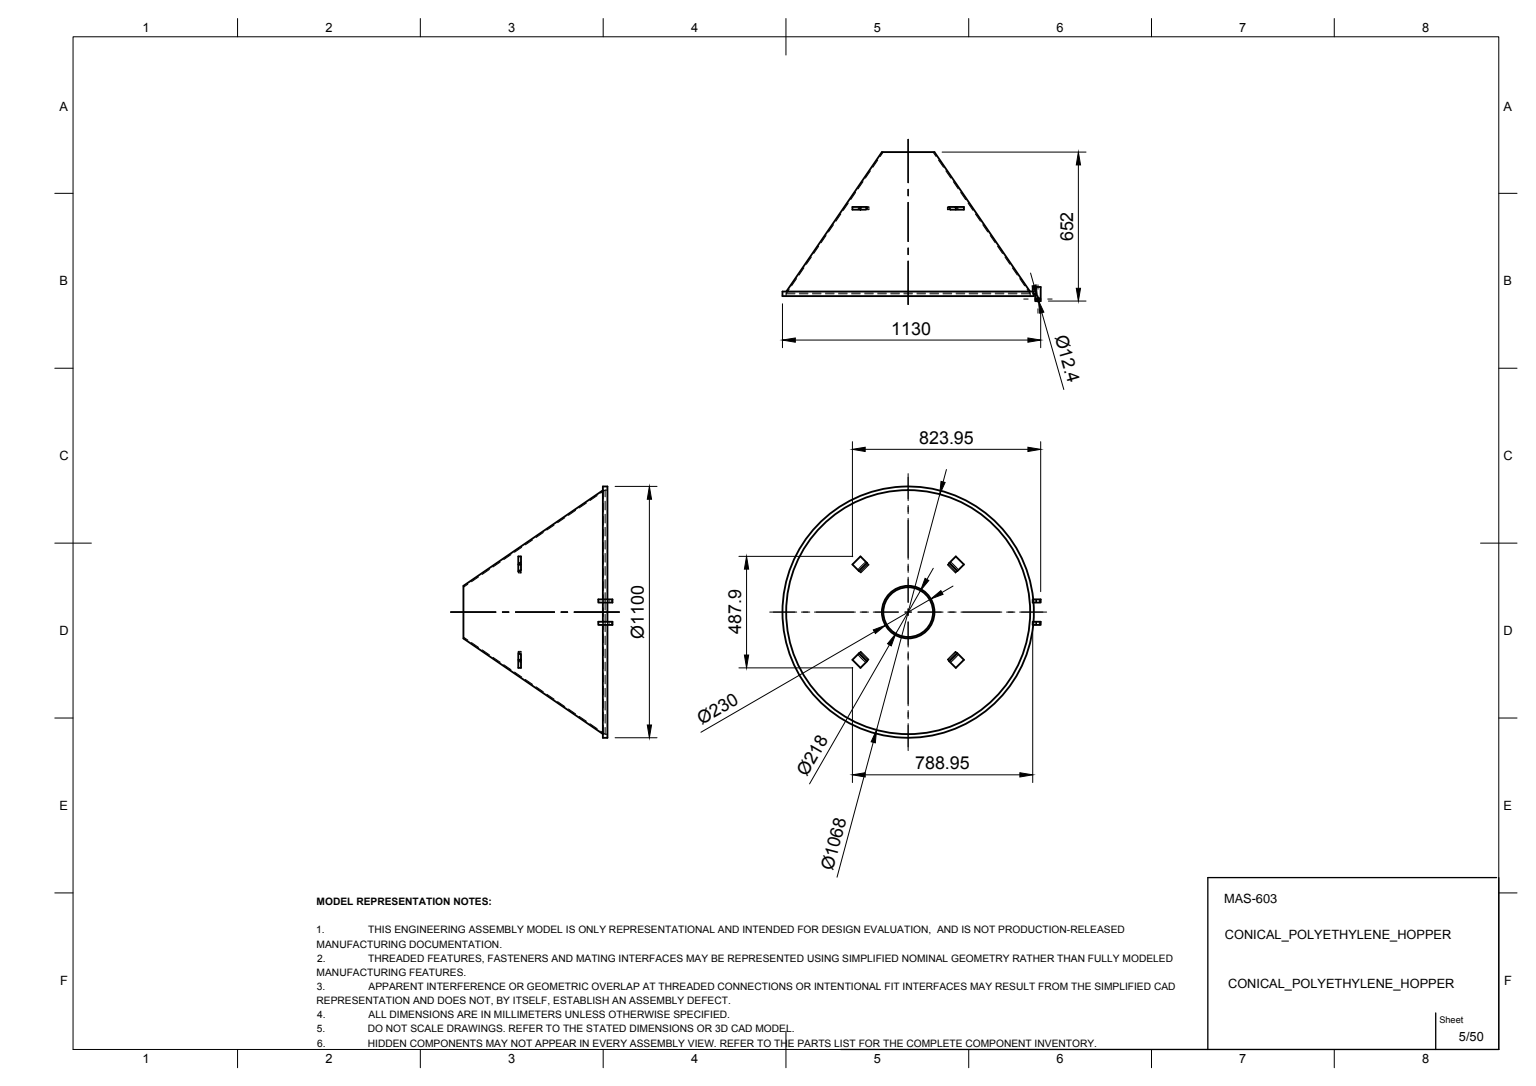
ISO-10303-21;
HEADER;
FILE_DESCRIPTION((''),'2;1');
FILE_NAME('CONICAL_POLYETHYLENE_HOPPER.step','2026-10-01T22:06:14-07:00',(''),(''),'','','');
FILE_SCHEMA (('AUTOMOTIVE_DESIGN { 1 0 10303 214 3 1 1 }'));
ENDSEC;
DATA;
#10=MECHANICAL_DESIGN_GEOMETRIC_PRESENTATION_REPRESENTATION('',(#981),#50440);
#891=SHAPE_REPRESENTATION_RELATIONSHIP('SRR','None',#50621,#936) ;
#936=ADVANCED_BREP_SHAPE_REPRESENTATION('',(#1037),#50390) ;
#981=STYLED_ITEM('',(#50884),#1037) ;
#1037=MANIFOLD_SOLID_BREP('CONICAL_POLYETHYLENE_HOPPER',#28629) ;
#1090=CONICAL_SURFACE('',#29307,32.15,0.600917014687121) ;
#1091=CONICAL_SURFACE('',#29309,32.75,0.600917014687121) ;
#1096=(
BOUNDED_CURVE()
B_SPLINE_CURVE(2,(#41351,#41352,#41353),.UNSPECIFIED.,.F.,.F.)
B_SPLINE_CURVE_WITH_KNOTS((3,3),(0.,1.45668740131038),.UNSPECIFIED.)
CURVE()
GEOMETRIC_REPRESENTATION_ITEM()
RATIONAL_B_SPLINE_CURVE((1.,1.00010597947028,1.))
REPRESENTATION_ITEM('')
) ;
#1097=(
BOUNDED_CURVE()
B_SPLINE_CURVE(2,(#41359,#41360,#41361),.UNSPECIFIED.,.F.,.F.)
B_SPLINE_CURVE_WITH_KNOTS((3,3),(0.,1.45668740131038),.UNSPECIFIED.)
CURVE()
GEOMETRIC_REPRESENTATION_ITEM()
RATIONAL_B_SPLINE_CURVE((1.,1.00010597945705,1.))
REPRESENTATION_ITEM('')
) ;
#1098=(
BOUNDED_CURVE()
B_SPLINE_CURVE(2,(#41368,#41369,#41370),.UNSPECIFIED.,.F.,.F.)
B_SPLINE_CURVE_WITH_KNOTS((3,3),(0.,1.45676753689758),.UNSPECIFIED.)
CURVE()
GEOMETRIC_REPRESENTATION_ITEM()
RATIONAL_B_SPLINE_CURVE((1.,1.00011064855622,1.))
REPRESENTATION_ITEM('')
) ;
#1099=(
BOUNDED_CURVE()
B_SPLINE_CURVE(2,(#41392,#41393,#41394),.UNSPECIFIED.,.F.,.F.)
B_SPLINE_CURVE_WITH_KNOTS((3,3),(0.,1.45676753689757),.UNSPECIFIED.)
CURVE()
GEOMETRIC_REPRESENTATION_ITEM()
RATIONAL_B_SPLINE_CURVE((1.,1.00011064897844,1.))
REPRESENTATION_ITEM('')
) ;
#1100=(
BOUNDED_CURVE()
B_SPLINE_CURVE(2,(#41409,#41410,#41411),.UNSPECIFIED.,.F.,.F.)
B_SPLINE_CURVE_WITH_KNOTS((3,3),(0.,1.45668740131038),.UNSPECIFIED.)
CURVE()
GEOMETRIC_REPRESENTATION_ITEM()
RATIONAL_B_SPLINE_CURVE((1.,1.00010597929787,1.))
REPRESENTATION_ITEM('')
) ;
#1101=(
BOUNDED_CURVE()
B_SPLINE_CURVE(2,(#41417,#41418,#41419),.UNSPECIFIED.,.F.,.F.)
B_SPLINE_CURVE_WITH_KNOTS((3,3),(0.,1.45668740131038),.UNSPECIFIED.)
CURVE()
GEOMETRIC_REPRESENTATION_ITEM()
RATIONAL_B_SPLINE_CURVE((1.,1.00010597985799,1.))
REPRESENTATION_ITEM('')
) ;
#1102=(
BOUNDED_CURVE()
B_SPLINE_CURVE(2,(#41426,#41427,#41428),.UNSPECIFIED.,.F.,.F.)
B_SPLINE_CURVE_WITH_KNOTS((3,3),(0.,1.45676753689758),.UNSPECIFIED.)
CURVE()
GEOMETRIC_REPRESENTATION_ITEM()
RATIONAL_B_SPLINE_CURVE((1.,1.00011064842347,1.))
REPRESENTATION_ITEM('')
) ;
#1103=(
BOUNDED_CURVE()
B_SPLINE_CURVE(2,(#41450,#41451,#41452),.UNSPECIFIED.,.F.,.F.)
B_SPLINE_CURVE_WITH_KNOTS((3,3),(0.,1.45676753689757),.UNSPECIFIED.)
CURVE()
GEOMETRIC_REPRESENTATION_ITEM()
RATIONAL_B_SPLINE_CURVE((1.,1.00011064825586,1.))
REPRESENTATION_ITEM('')
) ;
#1104=(
BOUNDED_CURVE()
B_SPLINE_CURVE(2,(#41467,#41468,#41469),.UNSPECIFIED.,.F.,.F.)
B_SPLINE_CURVE_WITH_KNOTS((3,3),(0.,1.45668740131038),.UNSPECIFIED.)
CURVE()
GEOMETRIC_REPRESENTATION_ITEM()
RATIONAL_B_SPLINE_CURVE((1.,1.00010597960991,1.))
REPRESENTATION_ITEM('')
) ;
#1105=(
BOUNDED_CURVE()
B_SPLINE_CURVE(2,(#41475,#41476,#41477),.UNSPECIFIED.,.F.,.F.)
B_SPLINE_CURVE_WITH_KNOTS((3,3),(0.,1.45668740131038),.UNSPECIFIED.)
CURVE()
GEOMETRIC_REPRESENTATION_ITEM()
RATIONAL_B_SPLINE_CURVE((1.,1.00010597917836,1.))
REPRESENTATION_ITEM('')
) ;
#1106=(
BOUNDED_CURVE()
B_SPLINE_CURVE(2,(#41484,#41485,#41486),.UNSPECIFIED.,.F.,.F.)
B_SPLINE_CURVE_WITH_KNOTS((3,3),(0.,1.45676753689757),.UNSPECIFIED.)
CURVE()
GEOMETRIC_REPRESENTATION_ITEM()
RATIONAL_B_SPLINE_CURVE((1.,1.00011064860079,1.))
REPRESENTATION_ITEM('')
) ;
#1107=(
BOUNDED_CURVE()
B_SPLINE_CURVE(2,(#41508,#41509,#41510),.UNSPECIFIED.,.F.,.F.)
B_SPLINE_CURVE_WITH_KNOTS((3,3),(0.,1.45676753689758),.UNSPECIFIED.)
CURVE()
GEOMETRIC_REPRESENTATION_ITEM()
RATIONAL_B_SPLINE_CURVE((1.,1.00011064816854,1.))
REPRESENTATION_ITEM('')
) ;
#1108=(
BOUNDED_CURVE()
B_SPLINE_CURVE(2,(#41525,#41526,#41527),.UNSPECIFIED.,.F.,.F.)
B_SPLINE_CURVE_WITH_KNOTS((3,3),(0.,1.45668740131038),.UNSPECIFIED.)
CURVE()
GEOMETRIC_REPRESENTATION_ITEM()
RATIONAL_B_SPLINE_CURVE((1.,1.00010597960991,1.))
REPRESENTATION_ITEM('')
) ;
#1109=(
BOUNDED_CURVE()
B_SPLINE_CURVE(2,(#41533,#41534,#41535),.UNSPECIFIED.,.F.,.F.)
B_SPLINE_CURVE_WITH_KNOTS((3,3),(0.,1.45668740131038),.UNSPECIFIED.)
CURVE()
GEOMETRIC_REPRESENTATION_ITEM()
RATIONAL_B_SPLINE_CURVE((1.,1.00010597917836,1.))
REPRESENTATION_ITEM('')
) ;
#1110=(
BOUNDED_CURVE()
B_SPLINE_CURVE(2,(#41542,#41543,#41544),.UNSPECIFIED.,.F.,.F.)
B_SPLINE_CURVE_WITH_KNOTS((3,3),(0.,1.45676753689757),.UNSPECIFIED.)
CURVE()
GEOMETRIC_REPRESENTATION_ITEM()
RATIONAL_B_SPLINE_CURVE((1.,1.00011064860079,1.))
REPRESENTATION_ITEM('')
) ;
#1111=(
BOUNDED_CURVE()
B_SPLINE_CURVE(2,(#41566,#41567,#41568),.UNSPECIFIED.,.F.,.F.)
B_SPLINE_CURVE_WITH_KNOTS((3,3),(0.,1.45676753689758),.UNSPECIFIED.)
CURVE()
GEOMETRIC_REPRESENTATION_ITEM()
RATIONAL_B_SPLINE_CURVE((1.,1.00011064816854,1.))
REPRESENTATION_ITEM('')
) ;
#1112=FACE_BOUND('',#3896,.T.) ;
#1113=FACE_BOUND('',#3903,.T.) ;
#1114=FACE_BOUND('',#3908,.T.) ;
#1115=FACE_BOUND('',#3915,.T.) ;
#1116=FACE_BOUND('',#3960,.T.) ;
#1117=FACE_BOUND('',#3962,.T.) ;
#1118=FACE_BOUND('',#3964,.T.) ;
#1119=FACE_BOUND('',#3965,.T.) ;
#1120=FACE_BOUND('',#3966,.T.) ;
#1121=FACE_BOUND('',#3967,.T.) ;
#1122=FACE_BOUND('',#3969,.T.) ;
#1123=FACE_BOUND('',#3970,.T.) ;
#1124=FACE_BOUND('',#3971,.T.) ;
#1125=FACE_BOUND('',#3972,.T.) ;
#1126=FACE_BOUND('',#3974,.T.) ;
#1408=PLANE('',#29217) ;
#1409=PLANE('',#29218) ;
#1410=PLANE('',#29219) ;
#1411=PLANE('',#29220) ;
#1412=PLANE('',#29221) ;
#1413=PLANE('',#29223) ;
#1414=PLANE('',#29224) ;
#1415=PLANE('',#29225) ;
#1416=PLANE('',#29235) ;
#1417=PLANE('',#29236) ;
#1418=PLANE('',#29237) ;
#1419=PLANE('',#29238) ;
#1420=PLANE('',#29239) ;
#1421=PLANE('',#29240) ;
#1422=PLANE('',#29241) ;
#1423=PLANE('',#29242) ;
#1424=PLANE('',#29243) ;
#1425=PLANE('',#29245) ;
#1426=PLANE('',#29246) ;
#1427=PLANE('',#29247) ;
#1428=PLANE('',#29248) ;
#1429=PLANE('',#29250) ;
#1430=PLANE('',#29252) ;
#1431=PLANE('',#29254) ;
#1432=PLANE('',#29255) ;
#1433=PLANE('',#29256) ;
#1434=PLANE('',#29257) ;
#1435=PLANE('',#29259) ;
#1436=PLANE('',#29260) ;
#1437=PLANE('',#29261) ;
#1438=PLANE('',#29262) ;
#1439=PLANE('',#29264) ;
#1440=PLANE('',#29266) ;
#1441=PLANE('',#29268) ;
#1442=PLANE('',#29269) ;
#1443=PLANE('',#29270) ;
#1444=PLANE('',#29271) ;
#1445=PLANE('',#29273) ;
#1446=PLANE('',#29274) ;
#1447=PLANE('',#29275) ;
#1448=PLANE('',#29276) ;
#1449=PLANE('',#29278) ;
#1450=PLANE('',#29280) ;
#1451=PLANE('',#29282) ;
#1452=PLANE('',#29283) ;
#1453=PLANE('',#29284) ;
#1454=PLANE('',#29285) ;
#1455=PLANE('',#29287) ;
#1456=PLANE('',#29288) ;
#1457=PLANE('',#29289) ;
#1458=PLANE('',#29290) ;
#1459=PLANE('',#29292) ;
#1460=PLANE('',#29294) ;
#1461=PLANE('',#29296) ;
#1462=PLANE('',#29297) ;
#1463=PLANE('',#29298) ;
#1464=PLANE('',#29305) ;
#1465=PLANE('',#29306) ;
#1466=PLANE('',#29311) ;
#2340=FACE_OUTER_BOUND('',#3894,.T.) ;
#2341=FACE_OUTER_BOUND('',#3895,.T.) ;
#2342=FACE_OUTER_BOUND('',#3897,.T.) ;
#2343=FACE_OUTER_BOUND('',#3898,.T.) ;
#2344=FACE_OUTER_BOUND('',#3899,.T.) ;
#2345=FACE_OUTER_BOUND('',#3900,.T.) ;
#2346=FACE_OUTER_BOUND('',#3901,.T.) ;
#2347=FACE_OUTER_BOUND('',#3902,.T.) ;
#2348=FACE_OUTER_BOUND('',#3904,.T.) ;
#2349=FACE_OUTER_BOUND('',#3905,.T.) ;
#2350=FACE_OUTER_BOUND('',#3906,.T.) ;
#2351=FACE_OUTER_BOUND('',#3907,.T.) ;
#2352=FACE_OUTER_BOUND('',#3909,.T.) ;
#2353=FACE_OUTER_BOUND('',#3910,.T.) ;
#2354=FACE_OUTER_BOUND('',#3911,.T.) ;
#2355=FACE_OUTER_BOUND('',#3912,.T.) ;
#2356=FACE_OUTER_BOUND('',#3913,.T.) ;
#2357=FACE_OUTER_BOUND('',#3914,.T.) ;
#2358=FACE_OUTER_BOUND('',#3916,.T.) ;
#2359=FACE_OUTER_BOUND('',#3917,.T.) ;
#2360=FACE_OUTER_BOUND('',#3918,.T.) ;
#2361=FACE_OUTER_BOUND('',#3919,.T.) ;
#2362=FACE_OUTER_BOUND('',#3920,.T.) ;
#2363=FACE_OUTER_BOUND('',#3921,.T.) ;
#2364=FACE_OUTER_BOUND('',#3922,.T.) ;
#2365=FACE_OUTER_BOUND('',#3923,.T.) ;
#2366=FACE_OUTER_BOUND('',#3924,.T.) ;
#2367=FACE_OUTER_BOUND('',#3925,.T.) ;
#2368=FACE_OUTER_BOUND('',#3926,.T.) ;
#2369=FACE_OUTER_BOUND('',#3927,.T.) ;
#2370=FACE_OUTER_BOUND('',#3928,.T.) ;
#2371=FACE_OUTER_BOUND('',#3929,.T.) ;
#2372=FACE_OUTER_BOUND('',#3930,.T.) ;
#2373=FACE_OUTER_BOUND('',#3931,.T.) ;
#2374=FACE_OUTER_BOUND('',#3932,.T.) ;
#2375=FACE_OUTER_BOUND('',#3933,.T.) ;
#2376=FACE_OUTER_BOUND('',#3934,.T.) ;
#2377=FACE_OUTER_BOUND('',#3935,.T.) ;
#2378=FACE_OUTER_BOUND('',#3936,.T.) ;
#2379=FACE_OUTER_BOUND('',#3937,.T.) ;
#2380=FACE_OUTER_BOUND('',#3938,.T.) ;
#2381=FACE_OUTER_BOUND('',#3939,.T.) ;
#2382=FACE_OUTER_BOUND('',#3940,.T.) ;
#2383=FACE_OUTER_BOUND('',#3941,.T.) ;
#2384=FACE_OUTER_BOUND('',#3942,.T.) ;
#2385=FACE_OUTER_BOUND('',#3943,.T.) ;
#2386=FACE_OUTER_BOUND('',#3944,.T.) ;
#2387=FACE_OUTER_BOUND('',#3945,.T.) ;
#2388=FACE_OUTER_BOUND('',#3946,.T.) ;
#2389=FACE_OUTER_BOUND('',#3947,.T.) ;
#2390=FACE_OUTER_BOUND('',#3948,.T.) ;
#2391=FACE_OUTER_BOUND('',#3949,.T.) ;
#2392=FACE_OUTER_BOUND('',#3950,.T.) ;
#2393=FACE_OUTER_BOUND('',#3951,.T.) ;
#2394=FACE_OUTER_BOUND('',#3952,.T.) ;
#2395=FACE_OUTER_BOUND('',#3953,.T.) ;
#2396=FACE_OUTER_BOUND('',#3954,.T.) ;
#2397=FACE_OUTER_BOUND('',#3955,.T.) ;
#2398=FACE_OUTER_BOUND('',#3956,.T.) ;
#2399=FACE_OUTER_BOUND('',#3957,.T.) ;
#2400=FACE_OUTER_BOUND('',#3958,.T.) ;
#2401=FACE_OUTER_BOUND('',#3959,.T.) ;
#2402=FACE_OUTER_BOUND('',#3961,.T.) ;
#2403=FACE_OUTER_BOUND('',#3963,.T.) ;
#2404=FACE_OUTER_BOUND('',#3968,.T.) ;
#2405=FACE_OUTER_BOUND('',#3973,.T.) ;
#3894=EDGE_LOOP('',(#18591,#18592,#18593,#18594)) ;
#3895=EDGE_LOOP('',(#18595,#18596,#18597,#18598,#18599,#18600,#18601,#18602)) ;
#3896=EDGE_LOOP('',(#18603)) ;
#3897=EDGE_LOOP('',(#18604,#18605,#18606,#18607)) ;
#3898=EDGE_LOOP('',(#18608,#18609,#18610,#18611)) ;
#3899=EDGE_LOOP('',(#18612,#18613,#18614,#18615)) ;
#3900=EDGE_LOOP('',(#18616,#18617,#18618,#18619)) ;
#3901=EDGE_LOOP('',(#18620,#18621,#18622,#18623)) ;
#3902=EDGE_LOOP('',(#18624,#18625,#18626,#18627,#18628,#18629,#18630,#18631)) ;
#3903=EDGE_LOOP('',(#18632)) ;
#3904=EDGE_LOOP('',(#18633,#18634,#18635,#18636)) ;
#3905=EDGE_LOOP('',(#18637,#18638,#18639,#18640,#18641,#18642,#18643,#18644,
#18645,#18646,#18647,#18648)) ;
#3906=EDGE_LOOP('',(#18649,#18650,#18651,#18652)) ;
#3907=EDGE_LOOP('',(#18653,#18654,#18655,#18656,#18657,#18658,#18659,#18660)) ;
#3908=EDGE_LOOP('',(#18661)) ;
#3909=EDGE_LOOP('',(#18662,#18663,#18664,#18665)) ;
#3910=EDGE_LOOP('',(#18666,#18667,#18668,#18669)) ;
#3911=EDGE_LOOP('',(#18670,#18671,#18672,#18673)) ;
#3912=EDGE_LOOP('',(#18674,#18675,#18676,#18677)) ;
#3913=EDGE_LOOP('',(#18678,#18679,#18680,#18681)) ;
#3914=EDGE_LOOP('',(#18682,#18683,#18684,#18685,#18686,#18687,#18688,#18689)) ;
#3915=EDGE_LOOP('',(#18690)) ;
#3916=EDGE_LOOP('',(#18691,#18692,#18693,#18694)) ;
#3917=EDGE_LOOP('',(#18695,#18696,#18697,#18698)) ;
#3918=EDGE_LOOP('',(#18699,#18700,#18701,#18702)) ;
#3919=EDGE_LOOP('',(#18703,#18704,#18705,#18706)) ;
#3920=EDGE_LOOP('',(#18707,#18708,#18709,#18710)) ;
#3921=EDGE_LOOP('',(#18711,#18712,#18713,#18714)) ;
#3922=EDGE_LOOP('',(#18715,#18716,#18717,#18718)) ;
#3923=EDGE_LOOP('',(#18719,#18720,#18721,#18722)) ;
#3924=EDGE_LOOP('',(#18723,#18724,#18725,#18726)) ;
#3925=EDGE_LOOP('',(#18727,#18728,#18729,#18730)) ;
#3926=EDGE_LOOP('',(#18731,#18732,#18733,#18734)) ;
#3927=EDGE_LOOP('',(#18735,#18736,#18737,#18738)) ;
#3928=EDGE_LOOP('',(#18739,#18740,#18741,#18742)) ;
#3929=EDGE_LOOP('',(#18743,#18744,#18745,#18746)) ;
#3930=EDGE_LOOP('',(#18747,#18748,#18749,#18750)) ;
#3931=EDGE_LOOP('',(#18751,#18752,#18753,#18754)) ;
#3932=EDGE_LOOP('',(#18755,#18756,#18757,#18758)) ;
#3933=EDGE_LOOP('',(#18759,#18760,#18761,#18762)) ;
#3934=EDGE_LOOP('',(#18763,#18764,#18765,#18766)) ;
#3935=EDGE_LOOP('',(#18767,#18768,#18769,#18770)) ;
#3936=EDGE_LOOP('',(#18771,#18772,#18773,#18774)) ;
#3937=EDGE_LOOP('',(#18775,#18776,#18777,#18778)) ;
#3938=EDGE_LOOP('',(#18779,#18780,#18781,#18782)) ;
#3939=EDGE_LOOP('',(#18783,#18784,#18785,#18786)) ;
#3940=EDGE_LOOP('',(#18787,#18788,#18789,#18790)) ;
#3941=EDGE_LOOP('',(#18791,#18792,#18793,#18794)) ;
#3942=EDGE_LOOP('',(#18795,#18796,#18797,#18798)) ;
#3943=EDGE_LOOP('',(#18799,#18800,#18801,#18802)) ;
#3944=EDGE_LOOP('',(#18803,#18804,#18805,#18806)) ;
#3945=EDGE_LOOP('',(#18807,#18808,#18809,#18810)) ;
#3946=EDGE_LOOP('',(#18811,#18812,#18813,#18814)) ;
#3947=EDGE_LOOP('',(#18815,#18816,#18817,#18818)) ;
#3948=EDGE_LOOP('',(#18819,#18820,#18821,#18822)) ;
#3949=EDGE_LOOP('',(#18823,#18824,#18825,#18826)) ;
#3950=EDGE_LOOP('',(#18827,#18828,#18829,#18830)) ;
#3951=EDGE_LOOP('',(#18831,#18832,#18833,#18834)) ;
#3952=EDGE_LOOP('',(#18835,#18836,#18837,#18838)) ;
#3953=EDGE_LOOP('',(#18839,#18840,#18841,#18842)) ;
#3954=EDGE_LOOP('',(#18843,#18844,#18845,#18846)) ;
#3955=EDGE_LOOP('',(#18847,#18848,#18849,#18850)) ;
#3956=EDGE_LOOP('',(#18851,#18852,#18853,#18854)) ;
#3957=EDGE_LOOP('',(#18855,#18856,#18857,#18858)) ;
#3958=EDGE_LOOP('',(#18859,#18860,#18861,#18862)) ;
#3959=EDGE_LOOP('',(#18863,#18864,#18865,#18866,#18867,#18868,#18869,#18870,
#18871)) ;
#3960=EDGE_LOOP('',(#18872)) ;
#3961=EDGE_LOOP('',(#18873)) ;
#3962=EDGE_LOOP('',(#18874)) ;
#3963=EDGE_LOOP('',(#18875,#18876,#18877,#18878)) ;
#3964=EDGE_LOOP('',(#18879,#18880,#18881,#18882)) ;
#3965=EDGE_LOOP('',(#18883,#18884,#18885,#18886)) ;
#3966=EDGE_LOOP('',(#18887,#18888,#18889,#18890)) ;
#3967=EDGE_LOOP('',(#18891,#18892,#18893,#18894)) ;
#3968=EDGE_LOOP('',(#18895,#18896,#18897,#18898)) ;
#3969=EDGE_LOOP('',(#18899,#18900,#18901,#18902)) ;
#3970=EDGE_LOOP('',(#18903,#18904,#18905,#18906)) ;
#3971=EDGE_LOOP('',(#18907,#18908,#18909,#18910)) ;
#3972=EDGE_LOOP('',(#18911,#18912,#18913,#18914)) ;
#3973=EDGE_LOOP('',(#18915)) ;
#3974=EDGE_LOOP('',(#18916)) ;
#5744=LINE('',#41230,#8216) ;
#5745=LINE('',#41235,#8217) ;
#5746=LINE('',#41237,#8218) ;
#5747=LINE('',#41239,#8219) ;
#5748=LINE('',#41241,#8220) ;
#5749=LINE('',#41243,#8221) ;
#5750=LINE('',#41245,#8222) ;
#5751=LINE('',#41247,#8223) ;
#5752=LINE('',#41248,#8224) ;
#5753=LINE('',#41251,#8225) ;
#5754=LINE('',#41253,#8226) ;
#5755=LINE('',#41254,#8227) ;
#5756=LINE('',#41257,#8228) ;
#5757=LINE('',#41259,#8229) ;
#5758=LINE('',#41260,#8230) ;
#5759=LINE('',#41263,#8231) ;
#5760=LINE('',#41264,#8232) ;
#5761=LINE('',#41268,#8233) ;
#5762=LINE('',#41271,#8234) ;
#5763=LINE('',#41272,#8235) ;
#5764=LINE('',#41275,#8236) ;
#5765=LINE('',#41276,#8237) ;
#5766=LINE('',#41277,#8238) ;
#5767=LINE('',#41283,#8239) ;
#5768=LINE('',#41287,#8240) ;
#5769=LINE('',#41291,#8241) ;
#5770=LINE('',#41298,#8242) ;
#5771=LINE('',#41302,#8243) ;
#5772=LINE('',#41304,#8244) ;
#5773=LINE('',#41306,#8245) ;
#5774=LINE('',#41308,#8246) ;
#5775=LINE('',#41310,#8247) ;
#5776=LINE('',#41312,#8248) ;
#5777=LINE('',#41313,#8249) ;
#5778=LINE('',#41316,#8250) ;
#5779=LINE('',#41318,#8251) ;
#5780=LINE('',#41319,#8252) ;
#5781=LINE('',#41322,#8253) ;
#5782=LINE('',#41324,#8254) ;
#5783=LINE('',#41325,#8255) ;
#5784=LINE('',#41328,#8256) ;
#5785=LINE('',#41329,#8257) ;
#5786=LINE('',#41331,#8258) ;
#5787=LINE('',#41334,#8259) ;
#5788=LINE('',#41335,#8260) ;
#5789=LINE('',#41337,#8261) ;
#5790=LINE('',#41338,#8262) ;
#5791=LINE('',#41345,#8263) ;
#5792=LINE('',#41347,#8264) ;
#5793=LINE('',#41348,#8265) ;
#5794=LINE('',#41355,#8266) ;
#5795=LINE('',#41356,#8267) ;
#5796=LINE('',#41363,#8268) ;
#5797=LINE('',#41364,#8269) ;
#5798=LINE('',#41372,#8270) ;
#5799=LINE('',#41374,#8271) ;
#5800=LINE('',#41375,#8272) ;
#5801=LINE('',#41378,#8273) ;
#5802=LINE('',#41383,#8274) ;
#5803=LINE('',#41384,#8275) ;
#5804=LINE('',#41389,#8276) ;
#5805=LINE('',#41390,#8277) ;
#5806=LINE('',#41395,#8278) ;
#5807=LINE('',#41403,#8279) ;
#5808=LINE('',#41405,#8280) ;
#5809=LINE('',#41406,#8281) ;
#5810=LINE('',#41413,#8282) ;
#5811=LINE('',#41414,#8283) ;
#5812=LINE('',#41421,#8284) ;
#5813=LINE('',#41422,#8285) ;
#5814=LINE('',#41430,#8286) ;
#5815=LINE('',#41432,#8287) ;
#5816=LINE('',#41433,#8288) ;
#5817=LINE('',#41436,#8289) ;
#5818=LINE('',#41441,#8290) ;
#5819=LINE('',#41442,#8291) ;
#5820=LINE('',#41447,#8292) ;
#5821=LINE('',#41448,#8293) ;
#5822=LINE('',#41453,#8294) ;
#5823=LINE('',#41461,#8295) ;
#5824=LINE('',#41463,#8296) ;
#5825=LINE('',#41464,#8297) ;
#5826=LINE('',#41471,#8298) ;
#5827=LINE('',#41472,#8299) ;
#5828=LINE('',#41479,#8300) ;
#5829=LINE('',#41480,#8301) ;
#5830=LINE('',#41488,#8302) ;
#5831=LINE('',#41490,#8303) ;
#5832=LINE('',#41491,#8304) ;
#5833=LINE('',#41494,#8305) ;
#5834=LINE('',#41499,#8306) ;
#5835=LINE('',#41500,#8307) ;
#5836=LINE('',#41505,#8308) ;
#5837=LINE('',#41506,#8309) ;
#5838=LINE('',#41511,#8310) ;
#5839=LINE('',#41519,#8311) ;
#5840=LINE('',#41521,#8312) ;
#5841=LINE('',#41522,#8313) ;
#5842=LINE('',#41529,#8314) ;
#5843=LINE('',#41530,#8315) ;
#5844=LINE('',#41537,#8316) ;
#5845=LINE('',#41538,#8317) ;
#5846=LINE('',#41546,#8318) ;
#5847=LINE('',#41548,#8319) ;
#5848=LINE('',#41549,#8320) ;
#5849=LINE('',#41552,#8321) ;
#5850=LINE('',#41557,#8322) ;
#5851=LINE('',#41558,#8323) ;
#5852=LINE('',#41563,#8324) ;
#5853=LINE('',#41564,#8325) ;
#5854=LINE('',#41569,#8326) ;
#5855=LINE('',#41576,#8327) ;
#5856=LINE('',#41582,#8328) ;
#5857=LINE('',#41589,#8329) ;
#5858=LINE('',#41592,#8330) ;
#8216=VECTOR('',#32401,0.62) ;
#8217=VECTOR('',#32406,1.) ;
#8218=VECTOR('',#32407,1.) ;
#8219=VECTOR('',#32408,1.) ;
#8220=VECTOR('',#32409,1.) ;
#8221=VECTOR('',#32410,1.) ;
#8222=VECTOR('',#32411,1.) ;
#8223=VECTOR('',#32412,1.) ;
#8224=VECTOR('',#32413,1.) ;
#8225=VECTOR('',#32416,1.) ;
#8226=VECTOR('',#32417,1.) ;
#8227=VECTOR('',#32418,1.) ;
#8228=VECTOR('',#32421,1.) ;
#8229=VECTOR('',#32422,1.) ;
#8230=VECTOR('',#32423,1.) ;
#8231=VECTOR('',#32426,1.) ;
#8232=VECTOR('',#32427,1.) ;
#8233=VECTOR('',#32432,1.) ;
#8234=VECTOR('',#32435,1.) ;
#8235=VECTOR('',#32436,1.) ;
#8236=VECTOR('',#32439,1.) ;
#8237=VECTOR('',#32440,1.) ;
#8238=VECTOR('',#32441,1.) ;
#8239=VECTOR('',#32448,55.) ;
#8240=VECTOR('',#32451,1.) ;
#8241=VECTOR('',#32454,1.) ;
#8242=VECTOR('',#32463,0.62) ;
#8243=VECTOR('',#32468,1.) ;
#8244=VECTOR('',#32469,1.) ;
#8245=VECTOR('',#32470,1.) ;
#8246=VECTOR('',#32471,1.) ;
#8247=VECTOR('',#32472,1.) ;
#8248=VECTOR('',#32473,1.) ;
#8249=VECTOR('',#32474,1.) ;
#8250=VECTOR('',#32477,1.) ;
#8251=VECTOR('',#32478,1.) ;
#8252=VECTOR('',#32479,1.) ;
#8253=VECTOR('',#32482,1.) ;
#8254=VECTOR('',#32483,1.) ;
#8255=VECTOR('',#32484,1.) ;
#8256=VECTOR('',#32487,1.) ;
#8257=VECTOR('',#32488,1.) ;
#8258=VECTOR('',#32491,1.) ;
#8259=VECTOR('',#32494,1.) ;
#8260=VECTOR('',#32495,1.) ;
#8261=VECTOR('',#32498,1.) ;
#8262=VECTOR('',#32499,1.) ;
#8263=VECTOR('',#32506,1.) ;
#8264=VECTOR('',#32507,1.) ;
#8265=VECTOR('',#32508,1.) ;
#8266=VECTOR('',#32511,1.) ;
#8267=VECTOR('',#32512,1.) ;
#8268=VECTOR('',#32515,1.) ;
#8269=VECTOR('',#32516,1.) ;
#8270=VECTOR('',#32519,1.) ;
#8271=VECTOR('',#32520,1.) ;
#8272=VECTOR('',#32521,1.) ;
#8273=VECTOR('',#32526,1.) ;
#8274=VECTOR('',#32531,1.) ;
#8275=VECTOR('',#32532,1.) ;
#8276=VECTOR('',#32537,1.) ;
#8277=VECTOR('',#32538,1.) ;
#8278=VECTOR('',#32541,1.) ;
#8279=VECTOR('',#32550,1.) ;
#8280=VECTOR('',#32551,1.) ;
#8281=VECTOR('',#32552,1.) ;
#8282=VECTOR('',#32555,1.) ;
#8283=VECTOR('',#32556,1.) ;
#8284=VECTOR('',#32559,1.) ;
#8285=VECTOR('',#32560,1.) ;
#8286=VECTOR('',#32563,1.) ;
#8287=VECTOR('',#32564,1.) ;
#8288=VECTOR('',#32565,1.) ;
#8289=VECTOR('',#32570,1.) ;
#8290=VECTOR('',#32575,1.) ;
#8291=VECTOR('',#32576,1.) ;
#8292=VECTOR('',#32581,1.) ;
#8293=VECTOR('',#32582,1.) ;
#8294=VECTOR('',#32585,1.) ;
#8295=VECTOR('',#32594,1.) ;
#8296=VECTOR('',#32595,1.) ;
#8297=VECTOR('',#32596,1.) ;
#8298=VECTOR('',#32599,1.) ;
#8299=VECTOR('',#32600,1.) ;
#8300=VECTOR('',#32603,1.) ;
#8301=VECTOR('',#32604,1.) ;
#8302=VECTOR('',#32607,1.) ;
#8303=VECTOR('',#32608,1.) ;
#8304=VECTOR('',#32609,1.) ;
#8305=VECTOR('',#32614,1.) ;
#8306=VECTOR('',#32619,1.) ;
#8307=VECTOR('',#32620,1.) ;
#8308=VECTOR('',#32625,1.) ;
#8309=VECTOR('',#32626,1.) ;
#8310=VECTOR('',#32629,1.) ;
#8311=VECTOR('',#32638,1.) ;
#8312=VECTOR('',#32639,1.) ;
#8313=VECTOR('',#32640,1.) ;
#8314=VECTOR('',#32643,1.) ;
#8315=VECTOR('',#32644,1.) ;
#8316=VECTOR('',#32647,1.) ;
#8317=VECTOR('',#32648,1.) ;
#8318=VECTOR('',#32651,1.) ;
#8319=VECTOR('',#32652,1.) ;
#8320=VECTOR('',#32653,1.) ;
#8321=VECTOR('',#32658,1.) ;
#8322=VECTOR('',#32663,1.) ;
#8323=VECTOR('',#32664,1.) ;
#8324=VECTOR('',#32669,1.) ;
#8325=VECTOR('',#32670,1.) ;
#8326=VECTOR('',#32673,1.) ;
#8327=VECTOR('',#32682,53.4) ;
#8328=VECTOR('',#32689,53.4) ;
#8329=VECTOR('',#32700,32.15) ;
#8330=VECTOR('',#32703,32.75) ;
#10688=CIRCLE('',#29215,0.62) ;
#10689=CIRCLE('',#29216,0.62) ;
#10690=CIRCLE('',#29222,55.) ;
#10691=CIRCLE('',#29227,55.) ;
#10692=CIRCLE('',#29228,55.) ;
#10693=CIRCLE('',#29229,55.) ;
#10694=CIRCLE('',#29230,55.) ;
#10695=CIRCLE('',#29231,55.) ;
#10696=CIRCLE('',#29233,0.62) ;
#10697=CIRCLE('',#29234,0.62) ;
#10698=CIRCLE('',#29244,28.7741935483871) ;
#10699=CIRCLE('',#29249,27.9516129032258) ;
#10700=CIRCLE('',#29251,27.3516129032258) ;
#10701=CIRCLE('',#29253,28.1741935483871) ;
#10702=CIRCLE('',#29258,28.7741935483871) ;
#10703=CIRCLE('',#29263,27.9516129032258) ;
#10704=CIRCLE('',#29265,27.3516129032258) ;
#10705=CIRCLE('',#29267,28.1741935483871) ;
#10706=CIRCLE('',#29272,28.7741935483871) ;
#10707=CIRCLE('',#29277,27.9516129032258) ;
#10708=CIRCLE('',#29279,27.3516129032258) ;
#10709=CIRCLE('',#29281,28.1741935483871) ;
#10710=CIRCLE('',#29286,28.7741935483871) ;
#10711=CIRCLE('',#29291,27.9516129032258) ;
#10712=CIRCLE('',#29293,27.3516129032258) ;
#10713=CIRCLE('',#29295,28.1741935483871) ;
#10714=CIRCLE('',#29300,53.4) ;
#10715=CIRCLE('',#29301,53.4) ;
#10716=CIRCLE('',#29303,53.4) ;
#10717=CIRCLE('',#29304,53.4) ;
#10718=CIRCLE('',#29308,10.9) ;
#10719=CIRCLE('',#29310,11.5) ;
#11855=VERTEX_POINT('',#41227) ;
#11856=VERTEX_POINT('',#41229) ;
#11857=VERTEX_POINT('',#41233) ;
#11858=VERTEX_POINT('',#41234) ;
#11859=VERTEX_POINT('',#41236) ;
#11860=VERTEX_POINT('',#41238) ;
#11861=VERTEX_POINT('',#41240) ;
#11862=VERTEX_POINT('',#41242) ;
#11863=VERTEX_POINT('',#41244) ;
#11864=VERTEX_POINT('',#41246) ;
#11865=VERTEX_POINT('',#41250) ;
#11866=VERTEX_POINT('',#41252) ;
#11867=VERTEX_POINT('',#41256) ;
#11868=VERTEX_POINT('',#41258) ;
#11869=VERTEX_POINT('',#41262) ;
#11870=VERTEX_POINT('',#41266) ;
#11871=VERTEX_POINT('',#41270) ;
#11872=VERTEX_POINT('',#41274) ;
#11873=VERTEX_POINT('',#41280) ;
#11874=VERTEX_POINT('',#41282) ;
#11875=VERTEX_POINT('',#41284) ;
#11876=VERTEX_POINT('',#41286) ;
#11877=VERTEX_POINT('',#41288) ;
#11878=VERTEX_POINT('',#41290) ;
#11879=VERTEX_POINT('',#41295) ;
#11880=VERTEX_POINT('',#41297) ;
#11881=VERTEX_POINT('',#41301) ;
#11882=VERTEX_POINT('',#41303) ;
#11883=VERTEX_POINT('',#41305) ;
#11884=VERTEX_POINT('',#41307) ;
#11885=VERTEX_POINT('',#41309) ;
#11886=VERTEX_POINT('',#41311) ;
#11887=VERTEX_POINT('',#41315) ;
#11888=VERTEX_POINT('',#41317) ;
#11889=VERTEX_POINT('',#41321) ;
#11890=VERTEX_POINT('',#41323) ;
#11891=VERTEX_POINT('',#41327) ;
#11892=VERTEX_POINT('',#41333) ;
#11893=VERTEX_POINT('',#41341) ;
#11894=VERTEX_POINT('',#41342) ;
#11895=VERTEX_POINT('',#41344) ;
#11896=VERTEX_POINT('',#41346) ;
#11897=VERTEX_POINT('',#41350) ;
#11898=VERTEX_POINT('',#41354) ;
#11899=VERTEX_POINT('',#41358) ;
#11900=VERTEX_POINT('',#41362) ;
#11901=VERTEX_POINT('',#41366) ;
#11902=VERTEX_POINT('',#41367) ;
#11903=VERTEX_POINT('',#41371) ;
#11904=VERTEX_POINT('',#41373) ;
#11905=VERTEX_POINT('',#41380) ;
#11906=VERTEX_POINT('',#41382) ;
#11907=VERTEX_POINT('',#41386) ;
#11908=VERTEX_POINT('',#41388) ;
#11909=VERTEX_POINT('',#41399) ;
#11910=VERTEX_POINT('',#41400) ;
#11911=VERTEX_POINT('',#41402) ;
#11912=VERTEX_POINT('',#41404) ;
#11913=VERTEX_POINT('',#41408) ;
#11914=VERTEX_POINT('',#41412) ;
#11915=VERTEX_POINT('',#41416) ;
#11916=VERTEX_POINT('',#41420) ;
#11917=VERTEX_POINT('',#41424) ;
#11918=VERTEX_POINT('',#41425) ;
#11919=VERTEX_POINT('',#41429) ;
#11920=VERTEX_POINT('',#41431) ;
#11921=VERTEX_POINT('',#41438) ;
#11922=VERTEX_POINT('',#41440) ;
#11923=VERTEX_POINT('',#41444) ;
#11924=VERTEX_POINT('',#41446) ;
#11925=VERTEX_POINT('',#41457) ;
#11926=VERTEX_POINT('',#41458) ;
#11927=VERTEX_POINT('',#41460) ;
#11928=VERTEX_POINT('',#41462) ;
#11929=VERTEX_POINT('',#41466) ;
#11930=VERTEX_POINT('',#41470) ;
#11931=VERTEX_POINT('',#41474) ;
#11932=VERTEX_POINT('',#41478) ;
#11933=VERTEX_POINT('',#41482) ;
#11934=VERTEX_POINT('',#41483) ;
#11935=VERTEX_POINT('',#41487) ;
#11936=VERTEX_POINT('',#41489) ;
#11937=VERTEX_POINT('',#41496) ;
#11938=VERTEX_POINT('',#41498) ;
#11939=VERTEX_POINT('',#41502) ;
#11940=VERTEX_POINT('',#41504) ;
#11941=VERTEX_POINT('',#41515) ;
#11942=VERTEX_POINT('',#41516) ;
#11943=VERTEX_POINT('',#41518) ;
#11944=VERTEX_POINT('',#41520) ;
#11945=VERTEX_POINT('',#41524) ;
#11946=VERTEX_POINT('',#41528) ;
#11947=VERTEX_POINT('',#41532) ;
#11948=VERTEX_POINT('',#41536) ;
#11949=VERTEX_POINT('',#41540) ;
#11950=VERTEX_POINT('',#41541) ;
#11951=VERTEX_POINT('',#41545) ;
#11952=VERTEX_POINT('',#41547) ;
#11953=VERTEX_POINT('',#41554) ;
#11954=VERTEX_POINT('',#41556) ;
#11955=VERTEX_POINT('',#41560) ;
#11956=VERTEX_POINT('',#41562) ;
#11957=VERTEX_POINT('',#41573) ;
#11958=VERTEX_POINT('',#41575) ;
#11959=VERTEX_POINT('',#41579) ;
#11960=VERTEX_POINT('',#41581) ;
#11961=VERTEX_POINT('',#41587) ;
#11962=VERTEX_POINT('',#41591) ;
#14561=EDGE_CURVE('',#11855,#11855,#10688,.T.) ;
#14562=EDGE_CURVE('',#11855,#11856,#5744,.T.) ;
#14563=EDGE_CURVE('',#11856,#11856,#10689,.T.) ;
#14564=EDGE_CURVE('',#11857,#11858,#5745,.T.) ;
#14565=EDGE_CURVE('',#11859,#11857,#5746,.T.) ;
#14566=EDGE_CURVE('',#11859,#11860,#5747,.T.) ;
#14567=EDGE_CURVE('',#11861,#11860,#5748,.T.) ;
#14568=EDGE_CURVE('',#11862,#11861,#5749,.T.) ;
#14569=EDGE_CURVE('',#11863,#11862,#5750,.T.) ;
#14570=EDGE_CURVE('',#11863,#11864,#5751,.T.) ;
#14571=EDGE_CURVE('',#11858,#11864,#5752,.T.) ;
#14572=EDGE_CURVE('',#11865,#11859,#5753,.T.) ;
#14573=EDGE_CURVE('',#11865,#11866,#5754,.T.) ;
#14574=EDGE_CURVE('',#11860,#11866,#5755,.T.) ;
#14575=EDGE_CURVE('',#11862,#11867,#5756,.T.) ;
#14576=EDGE_CURVE('',#11867,#11868,#5757,.T.) ;
#14577=EDGE_CURVE('',#11868,#11863,#5758,.T.) ;
#14578=EDGE_CURVE('',#11868,#11869,#5759,.T.) ;
#14579=EDGE_CURVE('',#11864,#11869,#5760,.T.) ;
#14580=EDGE_CURVE('',#11858,#11870,#10690,.T.) ;
#14581=EDGE_CURVE('',#11869,#11870,#5761,.T.) ;
#14582=EDGE_CURVE('',#11866,#11871,#5762,.T.) ;
#14583=EDGE_CURVE('',#11871,#11861,#5763,.T.) ;
#14584=EDGE_CURVE('',#11870,#11872,#5764,.T.) ;
#14585=EDGE_CURVE('',#11867,#11871,#5765,.T.) ;
#14586=EDGE_CURVE('',#11872,#11865,#5766,.T.) ;
#14587=EDGE_CURVE('',#11873,#11873,#10691,.T.) ;
#14588=EDGE_CURVE('',#11873,#11874,#5767,.T.) ;
#14589=EDGE_CURVE('',#11875,#11874,#10692,.T.) ;
#14590=EDGE_CURVE('',#11875,#11876,#5768,.T.) ;
#14591=EDGE_CURVE('',#11876,#11877,#10693,.T.) ;
#14592=EDGE_CURVE('',#11877,#11878,#5769,.T.) ;
#14593=EDGE_CURVE('',#11857,#11878,#10694,.T.) ;
#14594=EDGE_CURVE('',#11874,#11872,#10695,.T.) ;
#14595=EDGE_CURVE('',#11879,#11879,#10696,.T.) ;
#14596=EDGE_CURVE('',#11879,#11880,#5770,.T.) ;
#14597=EDGE_CURVE('',#11880,#11880,#10697,.T.) ;
#14598=EDGE_CURVE('',#11881,#11875,#5771,.T.) ;
#14599=EDGE_CURVE('',#11881,#11882,#5772,.T.) ;
#14600=EDGE_CURVE('',#11883,#11882,#5773,.T.) ;
#14601=EDGE_CURVE('',#11884,#11883,#5774,.T.) ;
#14602=EDGE_CURVE('',#11885,#11884,#5775,.T.) ;
#14603=EDGE_CURVE('',#11885,#11886,#5776,.T.) ;
#14604=EDGE_CURVE('',#11876,#11886,#5777,.T.) ;
#14605=EDGE_CURVE('',#11887,#11881,#5778,.T.) ;
#14606=EDGE_CURVE('',#11887,#11888,#5779,.T.) ;
#14607=EDGE_CURVE('',#11882,#11888,#5780,.T.) ;
#14608=EDGE_CURVE('',#11884,#11889,#5781,.T.) ;
#14609=EDGE_CURVE('',#11889,#11890,#5782,.T.) ;
#14610=EDGE_CURVE('',#11890,#11885,#5783,.T.) ;
#14611=EDGE_CURVE('',#11890,#11891,#5784,.T.) ;
#14612=EDGE_CURVE('',#11886,#11891,#5785,.T.) ;
#14613=EDGE_CURVE('',#11891,#11877,#5786,.T.) ;
#14614=EDGE_CURVE('',#11888,#11892,#5787,.T.) ;
#14615=EDGE_CURVE('',#11892,#11883,#5788,.T.) ;
#14616=EDGE_CURVE('',#11889,#11892,#5789,.T.) ;
#14617=EDGE_CURVE('',#11878,#11887,#5790,.T.) ;
#14618=EDGE_CURVE('',#11893,#11894,#10698,.T.) ;
#14619=EDGE_CURVE('',#11893,#11895,#5791,.T.) ;
#14620=EDGE_CURVE('',#11895,#11896,#5792,.T.) ;
#14621=EDGE_CURVE('',#11896,#11894,#5793,.T.) ;
#14622=EDGE_CURVE('',#11897,#11893,#1096,.T.) ;
#14623=EDGE_CURVE('',#11898,#11897,#5794,.T.) ;
#14624=EDGE_CURVE('',#11895,#11898,#5795,.T.) ;
#14625=EDGE_CURVE('',#11894,#11899,#1097,.T.) ;
#14626=EDGE_CURVE('',#11896,#11900,#5796,.T.) ;
#14627=EDGE_CURVE('',#11899,#11900,#5797,.T.) ;
#14628=EDGE_CURVE('',#11901,#11902,#1098,.T.) ;
#14629=EDGE_CURVE('',#11903,#11901,#5798,.T.) ;
#14630=EDGE_CURVE('',#11904,#11903,#5799,.T.) ;
#14631=EDGE_CURVE('',#11902,#11904,#5800,.T.) ;
#14632=EDGE_CURVE('',#11899,#11897,#10699,.T.) ;
#14633=EDGE_CURVE('',#11900,#11898,#5801,.T.) ;
#14634=EDGE_CURVE('',#11905,#11901,#10700,.T.) ;
#14635=EDGE_CURVE('',#11905,#11906,#5802,.T.) ;
#14636=EDGE_CURVE('',#11906,#11903,#5803,.T.) ;
#14637=EDGE_CURVE('',#11902,#11907,#10701,.T.) ;
#14638=EDGE_CURVE('',#11904,#11908,#5804,.T.) ;
#14639=EDGE_CURVE('',#11908,#11907,#5805,.T.) ;
#14640=EDGE_CURVE('',#11907,#11905,#1099,.T.) ;
#14641=EDGE_CURVE('',#11908,#11906,#5806,.T.) ;
#14642=EDGE_CURVE('',#11909,#11910,#10702,.T.) ;
#14643=EDGE_CURVE('',#11909,#11911,#5807,.T.) ;
#14644=EDGE_CURVE('',#11911,#11912,#5808,.T.) ;
#14645=EDGE_CURVE('',#11912,#11910,#5809,.T.) ;
#14646=EDGE_CURVE('',#11913,#11909,#1100,.T.) ;
#14647=EDGE_CURVE('',#11914,#11913,#5810,.T.) ;
#14648=EDGE_CURVE('',#11911,#11914,#5811,.T.) ;
#14649=EDGE_CURVE('',#11910,#11915,#1101,.T.) ;
#14650=EDGE_CURVE('',#11912,#11916,#5812,.T.) ;
#14651=EDGE_CURVE('',#11915,#11916,#5813,.T.) ;
#14652=EDGE_CURVE('',#11917,#11918,#1102,.T.) ;
#14653=EDGE_CURVE('',#11919,#11917,#5814,.T.) ;
#14654=EDGE_CURVE('',#11920,#11919,#5815,.T.) ;
#14655=EDGE_CURVE('',#11918,#11920,#5816,.T.) ;
#14656=EDGE_CURVE('',#11915,#11913,#10703,.T.) ;
#14657=EDGE_CURVE('',#11916,#11914,#5817,.T.) ;
#14658=EDGE_CURVE('',#11921,#11917,#10704,.T.) ;
#14659=EDGE_CURVE('',#11921,#11922,#5818,.T.) ;
#14660=EDGE_CURVE('',#11922,#11919,#5819,.T.) ;
#14661=EDGE_CURVE('',#11918,#11923,#10705,.T.) ;
#14662=EDGE_CURVE('',#11920,#11924,#5820,.T.) ;
#14663=EDGE_CURVE('',#11924,#11923,#5821,.T.) ;
#14664=EDGE_CURVE('',#11923,#11921,#1103,.T.) ;
#14665=EDGE_CURVE('',#11924,#11922,#5822,.T.) ;
#14666=EDGE_CURVE('',#11925,#11926,#10706,.T.) ;
#14667=EDGE_CURVE('',#11925,#11927,#5823,.T.) ;
#14668=EDGE_CURVE('',#11927,#11928,#5824,.T.) ;
#14669=EDGE_CURVE('',#11928,#11926,#5825,.T.) ;
#14670=EDGE_CURVE('',#11929,#11925,#1104,.T.) ;
#14671=EDGE_CURVE('',#11930,#11929,#5826,.T.) ;
#14672=EDGE_CURVE('',#11927,#11930,#5827,.T.) ;
#14673=EDGE_CURVE('',#11926,#11931,#1105,.T.) ;
#14674=EDGE_CURVE('',#11928,#11932,#5828,.T.) ;
#14675=EDGE_CURVE('',#11931,#11932,#5829,.T.) ;
#14676=EDGE_CURVE('',#11933,#11934,#1106,.T.) ;
#14677=EDGE_CURVE('',#11935,#11933,#5830,.T.) ;
#14678=EDGE_CURVE('',#11936,#11935,#5831,.T.) ;
#14679=EDGE_CURVE('',#11934,#11936,#5832,.T.) ;
#14680=EDGE_CURVE('',#11931,#11929,#10707,.T.) ;
#14681=EDGE_CURVE('',#11932,#11930,#5833,.T.) ;
#14682=EDGE_CURVE('',#11937,#11933,#10708,.T.) ;
#14683=EDGE_CURVE('',#11937,#11938,#5834,.T.) ;
#14684=EDGE_CURVE('',#11938,#11935,#5835,.T.) ;
#14685=EDGE_CURVE('',#11934,#11939,#10709,.T.) ;
#14686=EDGE_CURVE('',#11936,#11940,#5836,.T.) ;
#14687=EDGE_CURVE('',#11940,#11939,#5837,.T.) ;
#14688=EDGE_CURVE('',#11939,#11937,#1107,.T.) ;
#14689=EDGE_CURVE('',#11940,#11938,#5838,.T.) ;
#14690=EDGE_CURVE('',#11941,#11942,#10710,.T.) ;
#14691=EDGE_CURVE('',#11941,#11943,#5839,.T.) ;
#14692=EDGE_CURVE('',#11943,#11944,#5840,.T.) ;
#14693=EDGE_CURVE('',#11944,#11942,#5841,.T.) ;
#14694=EDGE_CURVE('',#11945,#11941,#1108,.T.) ;
#14695=EDGE_CURVE('',#11946,#11945,#5842,.T.) ;
#14696=EDGE_CURVE('',#11943,#11946,#5843,.T.) ;
#14697=EDGE_CURVE('',#11942,#11947,#1109,.T.) ;
#14698=EDGE_CURVE('',#11944,#11948,#5844,.T.) ;
#14699=EDGE_CURVE('',#11947,#11948,#5845,.T.) ;
#14700=EDGE_CURVE('',#11949,#11950,#1110,.T.) ;
#14701=EDGE_CURVE('',#11951,#11949,#5846,.T.) ;
#14702=EDGE_CURVE('',#11952,#11951,#5847,.T.) ;
#14703=EDGE_CURVE('',#11950,#11952,#5848,.T.) ;
#14704=EDGE_CURVE('',#11947,#11945,#10711,.T.) ;
#14705=EDGE_CURVE('',#11948,#11946,#5849,.T.) ;
#14706=EDGE_CURVE('',#11953,#11949,#10712,.T.) ;
#14707=EDGE_CURVE('',#11953,#11954,#5850,.T.) ;
#14708=EDGE_CURVE('',#11954,#11951,#5851,.T.) ;
#14709=EDGE_CURVE('',#11950,#11955,#10713,.T.) ;
#14710=EDGE_CURVE('',#11952,#11956,#5852,.T.) ;
#14711=EDGE_CURVE('',#11956,#11955,#5853,.T.) ;
#14712=EDGE_CURVE('',#11955,#11953,#1111,.T.) ;
#14713=EDGE_CURVE('',#11956,#11954,#5854,.T.) ;
#14714=EDGE_CURVE('',#11957,#11957,#10714,.T.) ;
#14715=EDGE_CURVE('',#11957,#11958,#5855,.T.) ;
#14716=EDGE_CURVE('',#11958,#11958,#10715,.T.) ;
#14717=EDGE_CURVE('',#11959,#11959,#10716,.T.) ;
#14718=EDGE_CURVE('',#11959,#11960,#5856,.T.) ;
#14719=EDGE_CURVE('',#11960,#11960,#10717,.T.) ;
#14720=EDGE_CURVE('',#11961,#11961,#10718,.T.) ;
#14721=EDGE_CURVE('',#11961,#11959,#5857,.T.) ;
#14722=EDGE_CURVE('',#11958,#11962,#5858,.T.) ;
#14723=EDGE_CURVE('',#11962,#11962,#10719,.T.) ;
#18591=ORIENTED_EDGE('',*,*,#14561,.F.) ;
#18592=ORIENTED_EDGE('',*,*,#14562,.T.) ;
#18593=ORIENTED_EDGE('',*,*,#14563,.F.) ;
#18594=ORIENTED_EDGE('',*,*,#14562,.F.) ;
#18595=ORIENTED_EDGE('',*,*,#14564,.F.) ;
#18596=ORIENTED_EDGE('',*,*,#14565,.F.) ;
#18597=ORIENTED_EDGE('',*,*,#14566,.T.) ;
#18598=ORIENTED_EDGE('',*,*,#14567,.F.) ;
#18599=ORIENTED_EDGE('',*,*,#14568,.F.) ;
#18600=ORIENTED_EDGE('',*,*,#14569,.F.) ;
#18601=ORIENTED_EDGE('',*,*,#14570,.T.) ;
#18602=ORIENTED_EDGE('',*,*,#14571,.F.) ;
#18603=ORIENTED_EDGE('',*,*,#14561,.T.) ;
#18604=ORIENTED_EDGE('',*,*,#14572,.F.) ;
#18605=ORIENTED_EDGE('',*,*,#14573,.T.) ;
#18606=ORIENTED_EDGE('',*,*,#14574,.F.) ;
#18607=ORIENTED_EDGE('',*,*,#14566,.F.) ;
#18608=ORIENTED_EDGE('',*,*,#14569,.T.) ;
#18609=ORIENTED_EDGE('',*,*,#14575,.T.) ;
#18610=ORIENTED_EDGE('',*,*,#14576,.T.) ;
#18611=ORIENTED_EDGE('',*,*,#14577,.T.) ;
#18612=ORIENTED_EDGE('',*,*,#14578,.T.) ;
#18613=ORIENTED_EDGE('',*,*,#14579,.F.) ;
#18614=ORIENTED_EDGE('',*,*,#14570,.F.) ;
#18615=ORIENTED_EDGE('',*,*,#14577,.F.) ;
#18616=ORIENTED_EDGE('',*,*,#14580,.F.) ;
#18617=ORIENTED_EDGE('',*,*,#14571,.T.) ;
#18618=ORIENTED_EDGE('',*,*,#14579,.T.) ;
#18619=ORIENTED_EDGE('',*,*,#14581,.T.) ;
#18620=ORIENTED_EDGE('',*,*,#14567,.T.) ;
#18621=ORIENTED_EDGE('',*,*,#14574,.T.) ;
#18622=ORIENTED_EDGE('',*,*,#14582,.T.) ;
#18623=ORIENTED_EDGE('',*,*,#14583,.T.) ;
#18624=ORIENTED_EDGE('',*,*,#14584,.F.) ;
#18625=ORIENTED_EDGE('',*,*,#14581,.F.) ;
#18626=ORIENTED_EDGE('',*,*,#14578,.F.) ;
#18627=ORIENTED_EDGE('',*,*,#14576,.F.) ;
#18628=ORIENTED_EDGE('',*,*,#14585,.T.) ;
#18629=ORIENTED_EDGE('',*,*,#14582,.F.) ;
#18630=ORIENTED_EDGE('',*,*,#14573,.F.) ;
#18631=ORIENTED_EDGE('',*,*,#14586,.F.) ;
#18632=ORIENTED_EDGE('',*,*,#14563,.T.) ;
#18633=ORIENTED_EDGE('',*,*,#14568,.T.) ;
#18634=ORIENTED_EDGE('',*,*,#14583,.F.) ;
#18635=ORIENTED_EDGE('',*,*,#14585,.F.) ;
#18636=ORIENTED_EDGE('',*,*,#14575,.F.) ;
#18637=ORIENTED_EDGE('',*,*,#14587,.F.) ;
#18638=ORIENTED_EDGE('',*,*,#14588,.T.) ;
#18639=ORIENTED_EDGE('',*,*,#14589,.F.) ;
#18640=ORIENTED_EDGE('',*,*,#14590,.T.) ;
#18641=ORIENTED_EDGE('',*,*,#14591,.T.) ;
#18642=ORIENTED_EDGE('',*,*,#14592,.T.) ;
#18643=ORIENTED_EDGE('',*,*,#14593,.F.) ;
#18644=ORIENTED_EDGE('',*,*,#14564,.T.) ;
#18645=ORIENTED_EDGE('',*,*,#14580,.T.) ;
#18646=ORIENTED_EDGE('',*,*,#14584,.T.) ;
#18647=ORIENTED_EDGE('',*,*,#14594,.F.) ;
#18648=ORIENTED_EDGE('',*,*,#14588,.F.) ;
#18649=ORIENTED_EDGE('',*,*,#14595,.F.) ;
#18650=ORIENTED_EDGE('',*,*,#14596,.T.) ;
#18651=ORIENTED_EDGE('',*,*,#14597,.F.) ;
#18652=ORIENTED_EDGE('',*,*,#14596,.F.) ;
#18653=ORIENTED_EDGE('',*,*,#14590,.F.) ;
#18654=ORIENTED_EDGE('',*,*,#14598,.F.) ;
#18655=ORIENTED_EDGE('',*,*,#14599,.T.) ;
#18656=ORIENTED_EDGE('',*,*,#14600,.F.) ;
#18657=ORIENTED_EDGE('',*,*,#14601,.F.) ;
#18658=ORIENTED_EDGE('',*,*,#14602,.F.) ;
#18659=ORIENTED_EDGE('',*,*,#14603,.T.) ;
#18660=ORIENTED_EDGE('',*,*,#14604,.F.) ;
#18661=ORIENTED_EDGE('',*,*,#14597,.T.) ;
#18662=ORIENTED_EDGE('',*,*,#14605,.F.) ;
#18663=ORIENTED_EDGE('',*,*,#14606,.T.) ;
#18664=ORIENTED_EDGE('',*,*,#14607,.F.) ;
#18665=ORIENTED_EDGE('',*,*,#14599,.F.) ;
#18666=ORIENTED_EDGE('',*,*,#14602,.T.) ;
#18667=ORIENTED_EDGE('',*,*,#14608,.T.) ;
#18668=ORIENTED_EDGE('',*,*,#14609,.T.) ;
#18669=ORIENTED_EDGE('',*,*,#14610,.T.) ;
#18670=ORIENTED_EDGE('',*,*,#14611,.T.) ;
#18671=ORIENTED_EDGE('',*,*,#14612,.F.) ;
#18672=ORIENTED_EDGE('',*,*,#14603,.F.) ;
#18673=ORIENTED_EDGE('',*,*,#14610,.F.) ;
#18674=ORIENTED_EDGE('',*,*,#14591,.F.) ;
#18675=ORIENTED_EDGE('',*,*,#14604,.T.) ;
#18676=ORIENTED_EDGE('',*,*,#14612,.T.) ;
#18677=ORIENTED_EDGE('',*,*,#14613,.T.) ;
#18678=ORIENTED_EDGE('',*,*,#14600,.T.) ;
#18679=ORIENTED_EDGE('',*,*,#14607,.T.) ;
#18680=ORIENTED_EDGE('',*,*,#14614,.T.) ;
#18681=ORIENTED_EDGE('',*,*,#14615,.T.) ;
#18682=ORIENTED_EDGE('',*,*,#14592,.F.) ;
#18683=ORIENTED_EDGE('',*,*,#14613,.F.) ;
#18684=ORIENTED_EDGE('',*,*,#14611,.F.) ;
#18685=ORIENTED_EDGE('',*,*,#14609,.F.) ;
#18686=ORIENTED_EDGE('',*,*,#14616,.T.) ;
#18687=ORIENTED_EDGE('',*,*,#14614,.F.) ;
#18688=ORIENTED_EDGE('',*,*,#14606,.F.) ;
#18689=ORIENTED_EDGE('',*,*,#14617,.F.) ;
#18690=ORIENTED_EDGE('',*,*,#14595,.T.) ;
#18691=ORIENTED_EDGE('',*,*,#14601,.T.) ;
#18692=ORIENTED_EDGE('',*,*,#14615,.F.) ;
#18693=ORIENTED_EDGE('',*,*,#14616,.F.) ;
#18694=ORIENTED_EDGE('',*,*,#14608,.F.) ;
#18695=ORIENTED_EDGE('',*,*,#14618,.F.) ;
#18696=ORIENTED_EDGE('',*,*,#14619,.T.) ;
#18697=ORIENTED_EDGE('',*,*,#14620,.T.) ;
#18698=ORIENTED_EDGE('',*,*,#14621,.T.) ;
#18699=ORIENTED_EDGE('',*,*,#14622,.F.) ;
#18700=ORIENTED_EDGE('',*,*,#14623,.F.) ;
#18701=ORIENTED_EDGE('',*,*,#14624,.F.) ;
#18702=ORIENTED_EDGE('',*,*,#14619,.F.) ;
#18703=ORIENTED_EDGE('',*,*,#14625,.F.) ;
#18704=ORIENTED_EDGE('',*,*,#14621,.F.) ;
#18705=ORIENTED_EDGE('',*,*,#14626,.T.) ;
#18706=ORIENTED_EDGE('',*,*,#14627,.F.) ;
#18707=ORIENTED_EDGE('',*,*,#14628,.F.) ;
#18708=ORIENTED_EDGE('',*,*,#14629,.F.) ;
#18709=ORIENTED_EDGE('',*,*,#14630,.F.) ;
#18710=ORIENTED_EDGE('',*,*,#14631,.F.) ;
#18711=ORIENTED_EDGE('',*,*,#14632,.F.) ;
#18712=ORIENTED_EDGE('',*,*,#14627,.T.) ;
#18713=ORIENTED_EDGE('',*,*,#14633,.T.) ;
#18714=ORIENTED_EDGE('',*,*,#14623,.T.) ;
#18715=ORIENTED_EDGE('',*,*,#14634,.F.) ;
#18716=ORIENTED_EDGE('',*,*,#14635,.T.) ;
#18717=ORIENTED_EDGE('',*,*,#14636,.T.) ;
#18718=ORIENTED_EDGE('',*,*,#14629,.T.) ;
#18719=ORIENTED_EDGE('',*,*,#14637,.F.) ;
#18720=ORIENTED_EDGE('',*,*,#14631,.T.) ;
#18721=ORIENTED_EDGE('',*,*,#14638,.T.) ;
#18722=ORIENTED_EDGE('',*,*,#14639,.T.) ;
#18723=ORIENTED_EDGE('',*,*,#14640,.F.) ;
#18724=ORIENTED_EDGE('',*,*,#14639,.F.) ;
#18725=ORIENTED_EDGE('',*,*,#14641,.T.) ;
#18726=ORIENTED_EDGE('',*,*,#14635,.F.) ;
#18727=ORIENTED_EDGE('',*,*,#14630,.T.) ;
#18728=ORIENTED_EDGE('',*,*,#14636,.F.) ;
#18729=ORIENTED_EDGE('',*,*,#14641,.F.) ;
#18730=ORIENTED_EDGE('',*,*,#14638,.F.) ;
#18731=ORIENTED_EDGE('',*,*,#14624,.T.) ;
#18732=ORIENTED_EDGE('',*,*,#14633,.F.) ;
#18733=ORIENTED_EDGE('',*,*,#14626,.F.) ;
#18734=ORIENTED_EDGE('',*,*,#14620,.F.) ;
#18735=ORIENTED_EDGE('',*,*,#14642,.F.) ;
#18736=ORIENTED_EDGE('',*,*,#14643,.T.) ;
#18737=ORIENTED_EDGE('',*,*,#14644,.T.) ;
#18738=ORIENTED_EDGE('',*,*,#14645,.T.) ;
#18739=ORIENTED_EDGE('',*,*,#14646,.F.) ;
#18740=ORIENTED_EDGE('',*,*,#14647,.F.) ;
#18741=ORIENTED_EDGE('',*,*,#14648,.F.) ;
#18742=ORIENTED_EDGE('',*,*,#14643,.F.) ;
#18743=ORIENTED_EDGE('',*,*,#14649,.F.) ;
#18744=ORIENTED_EDGE('',*,*,#14645,.F.) ;
#18745=ORIENTED_EDGE('',*,*,#14650,.T.) ;
#18746=ORIENTED_EDGE('',*,*,#14651,.F.) ;
#18747=ORIENTED_EDGE('',*,*,#14652,.F.) ;
#18748=ORIENTED_EDGE('',*,*,#14653,.F.) ;
#18749=ORIENTED_EDGE('',*,*,#14654,.F.) ;
#18750=ORIENTED_EDGE('',*,*,#14655,.F.) ;
#18751=ORIENTED_EDGE('',*,*,#14656,.F.) ;
#18752=ORIENTED_EDGE('',*,*,#14651,.T.) ;
#18753=ORIENTED_EDGE('',*,*,#14657,.T.) ;
#18754=ORIENTED_EDGE('',*,*,#14647,.T.) ;
#18755=ORIENTED_EDGE('',*,*,#14658,.F.) ;
#18756=ORIENTED_EDGE('',*,*,#14659,.T.) ;
#18757=ORIENTED_EDGE('',*,*,#14660,.T.) ;
#18758=ORIENTED_EDGE('',*,*,#14653,.T.) ;
#18759=ORIENTED_EDGE('',*,*,#14661,.F.) ;
#18760=ORIENTED_EDGE('',*,*,#14655,.T.) ;
#18761=ORIENTED_EDGE('',*,*,#14662,.T.) ;
#18762=ORIENTED_EDGE('',*,*,#14663,.T.) ;
#18763=ORIENTED_EDGE('',*,*,#14664,.F.) ;
#18764=ORIENTED_EDGE('',*,*,#14663,.F.) ;
#18765=ORIENTED_EDGE('',*,*,#14665,.T.) ;
#18766=ORIENTED_EDGE('',*,*,#14659,.F.) ;
#18767=ORIENTED_EDGE('',*,*,#14654,.T.) ;
#18768=ORIENTED_EDGE('',*,*,#14660,.F.) ;
#18769=ORIENTED_EDGE('',*,*,#14665,.F.) ;
#18770=ORIENTED_EDGE('',*,*,#14662,.F.) ;
#18771=ORIENTED_EDGE('',*,*,#14648,.T.) ;
#18772=ORIENTED_EDGE('',*,*,#14657,.F.) ;
#18773=ORIENTED_EDGE('',*,*,#14650,.F.) ;
#18774=ORIENTED_EDGE('',*,*,#14644,.F.) ;
#18775=ORIENTED_EDGE('',*,*,#14666,.F.) ;
#18776=ORIENTED_EDGE('',*,*,#14667,.T.) ;
#18777=ORIENTED_EDGE('',*,*,#14668,.T.) ;
#18778=ORIENTED_EDGE('',*,*,#14669,.T.) ;
#18779=ORIENTED_EDGE('',*,*,#14670,.F.) ;
#18780=ORIENTED_EDGE('',*,*,#14671,.F.) ;
#18781=ORIENTED_EDGE('',*,*,#14672,.F.) ;
#18782=ORIENTED_EDGE('',*,*,#14667,.F.) ;
#18783=ORIENTED_EDGE('',*,*,#14673,.F.) ;
#18784=ORIENTED_EDGE('',*,*,#14669,.F.) ;
#18785=ORIENTED_EDGE('',*,*,#14674,.T.) ;
#18786=ORIENTED_EDGE('',*,*,#14675,.F.) ;
#18787=ORIENTED_EDGE('',*,*,#14676,.F.) ;
#18788=ORIENTED_EDGE('',*,*,#14677,.F.) ;
#18789=ORIENTED_EDGE('',*,*,#14678,.F.) ;
#18790=ORIENTED_EDGE('',*,*,#14679,.F.) ;
#18791=ORIENTED_EDGE('',*,*,#14680,.F.) ;
#18792=ORIENTED_EDGE('',*,*,#14675,.T.) ;
#18793=ORIENTED_EDGE('',*,*,#14681,.T.) ;
#18794=ORIENTED_EDGE('',*,*,#14671,.T.) ;
#18795=ORIENTED_EDGE('',*,*,#14682,.F.) ;
#18796=ORIENTED_EDGE('',*,*,#14683,.T.) ;
#18797=ORIENTED_EDGE('',*,*,#14684,.T.) ;
#18798=ORIENTED_EDGE('',*,*,#14677,.T.) ;
#18799=ORIENTED_EDGE('',*,*,#14685,.F.) ;
#18800=ORIENTED_EDGE('',*,*,#14679,.T.) ;
#18801=ORIENTED_EDGE('',*,*,#14686,.T.) ;
#18802=ORIENTED_EDGE('',*,*,#14687,.T.) ;
#18803=ORIENTED_EDGE('',*,*,#14688,.F.) ;
#18804=ORIENTED_EDGE('',*,*,#14687,.F.) ;
#18805=ORIENTED_EDGE('',*,*,#14689,.T.) ;
#18806=ORIENTED_EDGE('',*,*,#14683,.F.) ;
#18807=ORIENTED_EDGE('',*,*,#14678,.T.) ;
#18808=ORIENTED_EDGE('',*,*,#14684,.F.) ;
#18809=ORIENTED_EDGE('',*,*,#14689,.F.) ;
#18810=ORIENTED_EDGE('',*,*,#14686,.F.) ;
#18811=ORIENTED_EDGE('',*,*,#14672,.T.) ;
#18812=ORIENTED_EDGE('',*,*,#14681,.F.) ;
#18813=ORIENTED_EDGE('',*,*,#14674,.F.) ;
#18814=ORIENTED_EDGE('',*,*,#14668,.F.) ;
#18815=ORIENTED_EDGE('',*,*,#14690,.F.) ;
#18816=ORIENTED_EDGE('',*,*,#14691,.T.) ;
#18817=ORIENTED_EDGE('',*,*,#14692,.T.) ;
#18818=ORIENTED_EDGE('',*,*,#14693,.T.) ;
#18819=ORIENTED_EDGE('',*,*,#14694,.F.) ;
#18820=ORIENTED_EDGE('',*,*,#14695,.F.) ;
#18821=ORIENTED_EDGE('',*,*,#14696,.F.) ;
#18822=ORIENTED_EDGE('',*,*,#14691,.F.) ;
#18823=ORIENTED_EDGE('',*,*,#14697,.F.) ;
#18824=ORIENTED_EDGE('',*,*,#14693,.F.) ;
#18825=ORIENTED_EDGE('',*,*,#14698,.T.) ;
#18826=ORIENTED_EDGE('',*,*,#14699,.F.) ;
#18827=ORIENTED_EDGE('',*,*,#14700,.F.) ;
#18828=ORIENTED_EDGE('',*,*,#14701,.F.) ;
#18829=ORIENTED_EDGE('',*,*,#14702,.F.) ;
#18830=ORIENTED_EDGE('',*,*,#14703,.F.) ;
#18831=ORIENTED_EDGE('',*,*,#14704,.F.) ;
#18832=ORIENTED_EDGE('',*,*,#14699,.T.) ;
#18833=ORIENTED_EDGE('',*,*,#14705,.T.) ;
#18834=ORIENTED_EDGE('',*,*,#14695,.T.) ;
#18835=ORIENTED_EDGE('',*,*,#14706,.F.) ;
#18836=ORIENTED_EDGE('',*,*,#14707,.T.) ;
#18837=ORIENTED_EDGE('',*,*,#14708,.T.) ;
#18838=ORIENTED_EDGE('',*,*,#14701,.T.) ;
#18839=ORIENTED_EDGE('',*,*,#14709,.F.) ;
#18840=ORIENTED_EDGE('',*,*,#14703,.T.) ;
#18841=ORIENTED_EDGE('',*,*,#14710,.T.) ;
#18842=ORIENTED_EDGE('',*,*,#14711,.T.) ;
#18843=ORIENTED_EDGE('',*,*,#14712,.F.) ;
#18844=ORIENTED_EDGE('',*,*,#14711,.F.) ;
#18845=ORIENTED_EDGE('',*,*,#14713,.T.) ;
#18846=ORIENTED_EDGE('',*,*,#14707,.F.) ;
#18847=ORIENTED_EDGE('',*,*,#14702,.T.) ;
#18848=ORIENTED_EDGE('',*,*,#14708,.F.) ;
#18849=ORIENTED_EDGE('',*,*,#14713,.F.) ;
#18850=ORIENTED_EDGE('',*,*,#14710,.F.) ;
#18851=ORIENTED_EDGE('',*,*,#14696,.T.) ;
#18852=ORIENTED_EDGE('',*,*,#14705,.F.) ;
#18853=ORIENTED_EDGE('',*,*,#14698,.F.) ;
#18854=ORIENTED_EDGE('',*,*,#14692,.F.) ;
#18855=ORIENTED_EDGE('',*,*,#14714,.F.) ;
#18856=ORIENTED_EDGE('',*,*,#14715,.T.) ;
#18857=ORIENTED_EDGE('',*,*,#14716,.F.) ;
#18858=ORIENTED_EDGE('',*,*,#14715,.F.) ;
#18859=ORIENTED_EDGE('',*,*,#14717,.T.) ;
#18860=ORIENTED_EDGE('',*,*,#14718,.T.) ;
#18861=ORIENTED_EDGE('',*,*,#14719,.F.) ;
#18862=ORIENTED_EDGE('',*,*,#14718,.F.) ;
#18863=ORIENTED_EDGE('',*,*,#14565,.T.) ;
#18864=ORIENTED_EDGE('',*,*,#14593,.T.) ;
#18865=ORIENTED_EDGE('',*,*,#14617,.T.) ;
#18866=ORIENTED_EDGE('',*,*,#14605,.T.) ;
#18867=ORIENTED_EDGE('',*,*,#14598,.T.) ;
#18868=ORIENTED_EDGE('',*,*,#14589,.T.) ;
#18869=ORIENTED_EDGE('',*,*,#14594,.T.) ;
#18870=ORIENTED_EDGE('',*,*,#14586,.T.) ;
#18871=ORIENTED_EDGE('',*,*,#14572,.T.) ;
#18872=ORIENTED_EDGE('',*,*,#14714,.T.) ;
#18873=ORIENTED_EDGE('',*,*,#14587,.T.) ;
#18874=ORIENTED_EDGE('',*,*,#14719,.T.) ;
#18875=ORIENTED_EDGE('',*,*,#14720,.F.) ;
#18876=ORIENTED_EDGE('',*,*,#14721,.T.) ;
#18877=ORIENTED_EDGE('',*,*,#14717,.F.) ;
#18878=ORIENTED_EDGE('',*,*,#14721,.F.) ;
#18879=ORIENTED_EDGE('',*,*,#14634,.T.) ;
#18880=ORIENTED_EDGE('',*,*,#14628,.T.) ;
#18881=ORIENTED_EDGE('',*,*,#14637,.T.) ;
#18882=ORIENTED_EDGE('',*,*,#14640,.T.) ;
#18883=ORIENTED_EDGE('',*,*,#14658,.T.) ;
#18884=ORIENTED_EDGE('',*,*,#14652,.T.) ;
#18885=ORIENTED_EDGE('',*,*,#14661,.T.) ;
#18886=ORIENTED_EDGE('',*,*,#14664,.T.) ;
#18887=ORIENTED_EDGE('',*,*,#14682,.T.) ;
#18888=ORIENTED_EDGE('',*,*,#14676,.T.) ;
#18889=ORIENTED_EDGE('',*,*,#14685,.T.) ;
#18890=ORIENTED_EDGE('',*,*,#14688,.T.) ;
#18891=ORIENTED_EDGE('',*,*,#14706,.T.) ;
#18892=ORIENTED_EDGE('',*,*,#14700,.T.) ;
#18893=ORIENTED_EDGE('',*,*,#14709,.T.) ;
#18894=ORIENTED_EDGE('',*,*,#14712,.T.) ;
#18895=ORIENTED_EDGE('',*,*,#14716,.T.) ;
#18896=ORIENTED_EDGE('',*,*,#14722,.T.) ;
#18897=ORIENTED_EDGE('',*,*,#14723,.F.) ;
#18898=ORIENTED_EDGE('',*,*,#14722,.F.) ;
#18899=ORIENTED_EDGE('',*,*,#14632,.T.) ;
#18900=ORIENTED_EDGE('',*,*,#14622,.T.) ;
#18901=ORIENTED_EDGE('',*,*,#14618,.T.) ;
#18902=ORIENTED_EDGE('',*,*,#14625,.T.) ;
#18903=ORIENTED_EDGE('',*,*,#14656,.T.) ;
#18904=ORIENTED_EDGE('',*,*,#14646,.T.) ;
#18905=ORIENTED_EDGE('',*,*,#14642,.T.) ;
#18906=ORIENTED_EDGE('',*,*,#14649,.T.) ;
#18907=ORIENTED_EDGE('',*,*,#14680,.T.) ;
#18908=ORIENTED_EDGE('',*,*,#14670,.T.) ;
#18909=ORIENTED_EDGE('',*,*,#14666,.T.) ;
#18910=ORIENTED_EDGE('',*,*,#14673,.T.) ;
#18911=ORIENTED_EDGE('',*,*,#14704,.T.) ;
#18912=ORIENTED_EDGE('',*,*,#14694,.T.) ;
#18913=ORIENTED_EDGE('',*,*,#14690,.T.) ;
#18914=ORIENTED_EDGE('',*,*,#14697,.T.) ;
#18915=ORIENTED_EDGE('',*,*,#14723,.T.) ;
#18916=ORIENTED_EDGE('',*,*,#14720,.T.) ;
#26651=CYLINDRICAL_SURFACE('',#29214,0.62) ;
#26652=CYLINDRICAL_SURFACE('',#29226,55.) ;
#26653=CYLINDRICAL_SURFACE('',#29232,0.62) ;
#26654=CYLINDRICAL_SURFACE('',#29299,53.4) ;
#26655=CYLINDRICAL_SURFACE('',#29302,53.4) ;
#27075=ADVANCED_FACE('',(#2340),#26651,.F.) ;
#27076=ADVANCED_FACE('',(#2341,#1112),#1408,.F.) ;
#27077=ADVANCED_FACE('',(#2342),#1409,.F.) ;
#27078=ADVANCED_FACE('',(#2343),#1410,.T.) ;
#27079=ADVANCED_FACE('',(#2344),#1411,.F.) ;
#27080=ADVANCED_FACE('',(#2345),#1412,.T.) ;
#27081=ADVANCED_FACE('',(#2346),#1413,.F.) ;
#27082=ADVANCED_FACE('',(#2347,#1113),#1414,.F.) ;
#27083=ADVANCED_FACE('',(#2348),#1415,.F.) ;
#27084=ADVANCED_FACE('',(#2349),#26652,.T.) ;
#27085=ADVANCED_FACE('',(#2350),#26653,.F.) ;
#27086=ADVANCED_FACE('',(#2351,#1114),#1416,.F.) ;
#27087=ADVANCED_FACE('',(#2352),#1417,.F.) ;
#27088=ADVANCED_FACE('',(#2353),#1418,.T.) ;
#27089=ADVANCED_FACE('',(#2354),#1419,.F.) ;
#27090=ADVANCED_FACE('',(#2355),#1420,.T.) ;
#27091=ADVANCED_FACE('',(#2356),#1421,.F.) ;
#27092=ADVANCED_FACE('',(#2357,#1115),#1422,.F.) ;
#27093=ADVANCED_FACE('',(#2358),#1423,.F.) ;
#27094=ADVANCED_FACE('',(#2359),#1424,.T.) ;
#27095=ADVANCED_FACE('',(#2360),#1425,.F.) ;
#27096=ADVANCED_FACE('',(#2361),#1426,.F.) ;
#27097=ADVANCED_FACE('',(#2362),#1427,.F.) ;
#27098=ADVANCED_FACE('',(#2363),#1428,.F.) ;
#27099=ADVANCED_FACE('',(#2364),#1429,.F.) ;
#27100=ADVANCED_FACE('',(#2365),#1430,.T.) ;
#27101=ADVANCED_FACE('',(#2366),#1431,.F.) ;
#27102=ADVANCED_FACE('',(#2367),#1432,.F.) ;
#27103=ADVANCED_FACE('',(#2368),#1433,.F.) ;
#27104=ADVANCED_FACE('',(#2369),#1434,.T.) ;
#27105=ADVANCED_FACE('',(#2370),#1435,.F.) ;
#27106=ADVANCED_FACE('',(#2371),#1436,.F.) ;
#27107=ADVANCED_FACE('',(#2372),#1437,.F.) ;
#27108=ADVANCED_FACE('',(#2373),#1438,.F.) ;
#27109=ADVANCED_FACE('',(#2374),#1439,.F.) ;
#27110=ADVANCED_FACE('',(#2375),#1440,.T.) ;
#27111=ADVANCED_FACE('',(#2376),#1441,.F.) ;
#27112=ADVANCED_FACE('',(#2377),#1442,.F.) ;
#27113=ADVANCED_FACE('',(#2378),#1443,.F.) ;
#27114=ADVANCED_FACE('',(#2379),#1444,.T.) ;
#27115=ADVANCED_FACE('',(#2380),#1445,.F.) ;
#27116=ADVANCED_FACE('',(#2381),#1446,.F.) ;
#27117=ADVANCED_FACE('',(#2382),#1447,.F.) ;
#27118=ADVANCED_FACE('',(#2383),#1448,.F.) ;
#27119=ADVANCED_FACE('',(#2384),#1449,.F.) ;
#27120=ADVANCED_FACE('',(#2385),#1450,.T.) ;
#27121=ADVANCED_FACE('',(#2386),#1451,.F.) ;
#27122=ADVANCED_FACE('',(#2387),#1452,.F.) ;
#27123=ADVANCED_FACE('',(#2388),#1453,.F.) ;
#27124=ADVANCED_FACE('',(#2389),#1454,.T.) ;
#27125=ADVANCED_FACE('',(#2390),#1455,.F.) ;
#27126=ADVANCED_FACE('',(#2391),#1456,.F.) ;
#27127=ADVANCED_FACE('',(#2392),#1457,.F.) ;
#27128=ADVANCED_FACE('',(#2393),#1458,.F.) ;
#27129=ADVANCED_FACE('',(#2394),#1459,.F.) ;
#27130=ADVANCED_FACE('',(#2395),#1460,.T.) ;
#27131=ADVANCED_FACE('',(#2396),#1461,.F.) ;
#27132=ADVANCED_FACE('',(#2397),#1462,.F.) ;
#27133=ADVANCED_FACE('',(#2398),#1463,.F.) ;
#27134=ADVANCED_FACE('',(#2399),#26654,.F.) ;
#27135=ADVANCED_FACE('',(#2400),#26655,.F.) ;
#27136=ADVANCED_FACE('',(#2401,#1116),#1464,.T.) ;
#27137=ADVANCED_FACE('',(#2402,#1117),#1465,.T.) ;
#27138=ADVANCED_FACE('',(#2403,#1118,#1119,#1120,#1121),#1090,.F.) ;
#27139=ADVANCED_FACE('',(#2404,#1122,#1123,#1124,#1125),#1091,.T.) ;
#27140=ADVANCED_FACE('',(#2405,#1126),#1466,.T.) ;
#28629=CLOSED_SHELL('',(#27075,#27076,#27077,#27078,#27079,#27080,#27081,
#27082,#27083,#27084,#27085,#27086,#27087,#27088,#27089,#27090,#27091,#27092,
#27093,#27094,#27095,#27096,#27097,#27098,#27099,#27100,#27101,#27102,#27103,
#27104,#27105,#27106,#27107,#27108,#27109,#27110,#27111,#27112,#27113,#27114,
#27115,#27116,#27117,#27118,#27119,#27120,#27121,#27122,#27123,#27124,#27125,
#27126,#27127,#27128,#27129,#27130,#27131,#27132,#27133,#27134,#27135,#27136,
#27137,#27138,#27139,#27140)) ;
#29213=AXIS2_PLACEMENT_3D('',#41225,#32395,#32396) ;
#29214=AXIS2_PLACEMENT_3D('',#41226,#32397,#32398) ;
#29215=AXIS2_PLACEMENT_3D('',#41228,#32399,#32400) ;
#29216=AXIS2_PLACEMENT_3D('',#41231,#32402,#32403) ;
#29217=AXIS2_PLACEMENT_3D('',#41232,#32404,#32405) ;
#29218=AXIS2_PLACEMENT_3D('',#41249,#32414,#32415) ;
#29219=AXIS2_PLACEMENT_3D('',#41255,#32419,#32420) ;
#29220=AXIS2_PLACEMENT_3D('',#41261,#32424,#32425) ;
#29221=AXIS2_PLACEMENT_3D('',#41265,#32428,#32429) ;
#29222=AXIS2_PLACEMENT_3D('',#41267,#32430,#32431) ;
#29223=AXIS2_PLACEMENT_3D('',#41269,#32433,#32434) ;
#29224=AXIS2_PLACEMENT_3D('',#41273,#32437,#32438) ;
#29225=AXIS2_PLACEMENT_3D('',#41278,#32442,#32443) ;
#29226=AXIS2_PLACEMENT_3D('',#41279,#32444,#32445) ;
#29227=AXIS2_PLACEMENT_3D('',#41281,#32446,#32447) ;
#29228=AXIS2_PLACEMENT_3D('',#41285,#32449,#32450) ;
#29229=AXIS2_PLACEMENT_3D('',#41289,#32452,#32453) ;
#29230=AXIS2_PLACEMENT_3D('',#41292,#32455,#32456) ;
#29231=AXIS2_PLACEMENT_3D('',#41293,#32457,#32458) ;
#29232=AXIS2_PLACEMENT_3D('',#41294,#32459,#32460) ;
#29233=AXIS2_PLACEMENT_3D('',#41296,#32461,#32462) ;
#29234=AXIS2_PLACEMENT_3D('',#41299,#32464,#32465) ;
#29235=AXIS2_PLACEMENT_3D('',#41300,#32466,#32467) ;
#29236=AXIS2_PLACEMENT_3D('',#41314,#32475,#32476) ;
#29237=AXIS2_PLACEMENT_3D('',#41320,#32480,#32481) ;
#29238=AXIS2_PLACEMENT_3D('',#41326,#32485,#32486) ;
#29239=AXIS2_PLACEMENT_3D('',#41330,#32489,#32490) ;
#29240=AXIS2_PLACEMENT_3D('',#41332,#32492,#32493) ;
#29241=AXIS2_PLACEMENT_3D('',#41336,#32496,#32497) ;
#29242=AXIS2_PLACEMENT_3D('',#41339,#32500,#32501) ;
#29243=AXIS2_PLACEMENT_3D('',#41340,#32502,#32503) ;
#29244=AXIS2_PLACEMENT_3D('',#41343,#32504,#32505) ;
#29245=AXIS2_PLACEMENT_3D('',#41349,#32509,#32510) ;
#29246=AXIS2_PLACEMENT_3D('',#41357,#32513,#32514) ;
#29247=AXIS2_PLACEMENT_3D('',#41365,#32517,#32518) ;
#29248=AXIS2_PLACEMENT_3D('',#41376,#32522,#32523) ;
#29249=AXIS2_PLACEMENT_3D('',#41377,#32524,#32525) ;
#29250=AXIS2_PLACEMENT_3D('',#41379,#32527,#32528) ;
#29251=AXIS2_PLACEMENT_3D('',#41381,#32529,#32530) ;
#29252=AXIS2_PLACEMENT_3D('',#41385,#32533,#32534) ;
#29253=AXIS2_PLACEMENT_3D('',#41387,#32535,#32536) ;
#29254=AXIS2_PLACEMENT_3D('',#41391,#32539,#32540) ;
#29255=AXIS2_PLACEMENT_3D('',#41396,#32542,#32543) ;
#29256=AXIS2_PLACEMENT_3D('',#41397,#32544,#32545) ;
#29257=AXIS2_PLACEMENT_3D('',#41398,#32546,#32547) ;
#29258=AXIS2_PLACEMENT_3D('',#41401,#32548,#32549) ;
#29259=AXIS2_PLACEMENT_3D('',#41407,#32553,#32554) ;
#29260=AXIS2_PLACEMENT_3D('',#41415,#32557,#32558) ;
#29261=AXIS2_PLACEMENT_3D('',#41423,#32561,#32562) ;
#29262=AXIS2_PLACEMENT_3D('',#41434,#32566,#32567) ;
#29263=AXIS2_PLACEMENT_3D('',#41435,#32568,#32569) ;
#29264=AXIS2_PLACEMENT_3D('',#41437,#32571,#32572) ;
#29265=AXIS2_PLACEMENT_3D('',#41439,#32573,#32574) ;
#29266=AXIS2_PLACEMENT_3D('',#41443,#32577,#32578) ;
#29267=AXIS2_PLACEMENT_3D('',#41445,#32579,#32580) ;
#29268=AXIS2_PLACEMENT_3D('',#41449,#32583,#32584) ;
#29269=AXIS2_PLACEMENT_3D('',#41454,#32586,#32587) ;
#29270=AXIS2_PLACEMENT_3D('',#41455,#32588,#32589) ;
#29271=AXIS2_PLACEMENT_3D('',#41456,#32590,#32591) ;
#29272=AXIS2_PLACEMENT_3D('',#41459,#32592,#32593) ;
#29273=AXIS2_PLACEMENT_3D('',#41465,#32597,#32598) ;
#29274=AXIS2_PLACEMENT_3D('',#41473,#32601,#32602) ;
#29275=AXIS2_PLACEMENT_3D('',#41481,#32605,#32606) ;
#29276=AXIS2_PLACEMENT_3D('',#41492,#32610,#32611) ;
#29277=AXIS2_PLACEMENT_3D('',#41493,#32612,#32613) ;
#29278=AXIS2_PLACEMENT_3D('',#41495,#32615,#32616) ;
#29279=AXIS2_PLACEMENT_3D('',#41497,#32617,#32618) ;
#29280=AXIS2_PLACEMENT_3D('',#41501,#32621,#32622) ;
#29281=AXIS2_PLACEMENT_3D('',#41503,#32623,#32624) ;
#29282=AXIS2_PLACEMENT_3D('',#41507,#32627,#32628) ;
#29283=AXIS2_PLACEMENT_3D('',#41512,#32630,#32631) ;
#29284=AXIS2_PLACEMENT_3D('',#41513,#32632,#32633) ;
#29285=AXIS2_PLACEMENT_3D('',#41514,#32634,#32635) ;
#29286=AXIS2_PLACEMENT_3D('',#41517,#32636,#32637) ;
#29287=AXIS2_PLACEMENT_3D('',#41523,#32641,#32642) ;
#29288=AXIS2_PLACEMENT_3D('',#41531,#32645,#32646) ;
#29289=AXIS2_PLACEMENT_3D('',#41539,#32649,#32650) ;
#29290=AXIS2_PLACEMENT_3D('',#41550,#32654,#32655) ;
#29291=AXIS2_PLACEMENT_3D('',#41551,#32656,#32657) ;
#29292=AXIS2_PLACEMENT_3D('',#41553,#32659,#32660) ;
#29293=AXIS2_PLACEMENT_3D('',#41555,#32661,#32662) ;
#29294=AXIS2_PLACEMENT_3D('',#41559,#32665,#32666) ;
#29295=AXIS2_PLACEMENT_3D('',#41561,#32667,#32668) ;
#29296=AXIS2_PLACEMENT_3D('',#41565,#32671,#32672) ;
#29297=AXIS2_PLACEMENT_3D('',#41570,#32674,#32675) ;
#29298=AXIS2_PLACEMENT_3D('',#41571,#32676,#32677) ;
#29299=AXIS2_PLACEMENT_3D('',#41572,#32678,#32679) ;
#29300=AXIS2_PLACEMENT_3D('',#41574,#32680,#32681) ;
#29301=AXIS2_PLACEMENT_3D('',#41577,#32683,#32684) ;
#29302=AXIS2_PLACEMENT_3D('',#41578,#32685,#32686) ;
#29303=AXIS2_PLACEMENT_3D('',#41580,#32687,#32688) ;
#29304=AXIS2_PLACEMENT_3D('',#41583,#32690,#32691) ;
#29305=AXIS2_PLACEMENT_3D('',#41584,#32692,#32693) ;
#29306=AXIS2_PLACEMENT_3D('',#41585,#32694,#32695) ;
#29307=AXIS2_PLACEMENT_3D('',#41586,#32696,#32697) ;
#29308=AXIS2_PLACEMENT_3D('',#41588,#32698,#32699) ;
#29309=AXIS2_PLACEMENT_3D('',#41590,#32701,#32702) ;
#29310=AXIS2_PLACEMENT_3D('',#41593,#32704,#32705) ;
#29311=AXIS2_PLACEMENT_3D('',#41594,#32706,#32707) ;
#32395=DIRECTION('axis',(0.,0.,1.)) ;
#32396=DIRECTION('refdir',(1.,0.,0.)) ;
#32397=DIRECTION('center_axis',(-1.,0.,0.)) ;
#32398=DIRECTION('ref_axis',(0.,0.,1.)) ;
#32399=DIRECTION('center_axis',(-1.,0.,0.)) ;
#32400=DIRECTION('ref_axis',(0.,0.,1.)) ;
#32401=DIRECTION('',(-1.,0.,0.)) ;
#32402=DIRECTION('center_axis',(1.,0.,0.)) ;
#32403=DIRECTION('ref_axis',(0.,0.,1.)) ;
#32404=DIRECTION('center_axis',(-1.,0.,0.)) ;
#32405=DIRECTION('ref_axis',(0.,0.,1.)) ;
#32406=DIRECTION('',(0.,0.,1.)) ;
#32407=DIRECTION('',(0.,1.,0.)) ;
#32408=DIRECTION('',(0.,0.,-1.)) ;
#32409=DIRECTION('',(0.,-1.,0.)) ;
#32410=DIRECTION('',(0.,0.,-1.)) ;
#32411=DIRECTION('',(0.,1.,0.)) ;
#32412=DIRECTION('',(0.,0.,-1.)) ;
#32413=DIRECTION('',(0.,1.,0.)) ;
#32414=DIRECTION('center_axis',(0.,1.,0.)) ;
#32415=DIRECTION('ref_axis',(0.,0.,1.)) ;
#32416=DIRECTION('',(1.,0.,0.)) ;
#32417=DIRECTION('',(0.,0.,-1.)) ;
#32418=DIRECTION('',(-1.,0.,0.)) ;
#32419=DIRECTION('center_axis',(0.,0.,1.)) ;
#32420=DIRECTION('ref_axis',(1.,0.,0.)) ;
#32421=DIRECTION('',(-1.,0.,0.)) ;
#32422=DIRECTION('',(0.,-1.,0.)) ;
#32423=DIRECTION('',(1.,0.,0.)) ;
#32424=DIRECTION('center_axis',(0.,1.,0.)) ;
#32425=DIRECTION('ref_axis',(0.,0.,1.)) ;
#32426=DIRECTION('',(0.,0.,-1.)) ;
#32427=DIRECTION('',(-1.,0.,0.)) ;
#32428=DIRECTION('center_axis',(0.,0.,1.)) ;
#32429=DIRECTION('ref_axis',(1.,0.,0.)) ;
#32430=DIRECTION('center_axis',(0.,0.,1.)) ;
#32431=DIRECTION('ref_axis',(1.,0.,0.)) ;
#32432=DIRECTION('',(0.,-1.,0.)) ;
#32433=DIRECTION('center_axis',(0.,0.,1.)) ;
#32434=DIRECTION('ref_axis',(1.,0.,0.)) ;
#32435=DIRECTION('',(0.,1.,0.)) ;
#32436=DIRECTION('',(1.,0.,0.)) ;
#32437=DIRECTION('center_axis',(1.,0.,0.)) ;
#32438=DIRECTION('ref_axis',(0.,0.,-1.)) ;
#32439=DIRECTION('',(0.,0.,-1.)) ;
#32440=DIRECTION('',(0.,0.,-1.)) ;
#32441=DIRECTION('',(0.,-1.,0.)) ;
#32442=DIRECTION('center_axis',(0.,-1.,0.)) ;
#32443=DIRECTION('ref_axis',(0.,0.,-1.)) ;
#32444=DIRECTION('center_axis',(0.,0.,1.)) ;
#32445=DIRECTION('ref_axis',(1.,0.,0.)) ;
#32446=DIRECTION('center_axis',(0.,0.,1.)) ;
#32447=DIRECTION('ref_axis',(1.,0.,0.)) ;
#32448=DIRECTION('',(0.,0.,-1.)) ;
#32449=DIRECTION('center_axis',(0.,0.,-1.)) ;
#32450=DIRECTION('ref_axis',(1.,0.,0.)) ;
#32451=DIRECTION('',(0.,0.,1.)) ;
#32452=DIRECTION('center_axis',(0.,0.,1.)) ;
#32453=DIRECTION('ref_axis',(1.,0.,0.)) ;
#32454=DIRECTION('',(0.,0.,-1.)) ;
#32455=DIRECTION('center_axis',(0.,0.,-1.)) ;
#32456=DIRECTION('ref_axis',(1.,0.,0.)) ;
#32457=DIRECTION('center_axis',(0.,0.,-1.)) ;
#32458=DIRECTION('ref_axis',(1.,0.,0.)) ;
#32459=DIRECTION('center_axis',(1.,0.,0.)) ;
#32460=DIRECTION('ref_axis',(0.,0.,-1.)) ;
#32461=DIRECTION('center_axis',(1.,0.,0.)) ;
#32462=DIRECTION('ref_axis',(0.,0.,-1.)) ;
#32463=DIRECTION('',(1.,0.,0.)) ;
#32464=DIRECTION('center_axis',(-1.,0.,0.)) ;
#32465=DIRECTION('ref_axis',(0.,0.,-1.)) ;
#32466=DIRECTION('center_axis',(-1.,0.,0.)) ;
#32467=DIRECTION('ref_axis',(0.,0.,1.)) ;
#32468=DIRECTION('',(0.,1.,0.)) ;
#32469=DIRECTION('',(0.,0.,-1.)) ;
#32470=DIRECTION('',(0.,-1.,0.)) ;
#32471=DIRECTION('',(0.,0.,-1.)) ;
#32472=DIRECTION('',(0.,1.,0.)) ;
#32473=DIRECTION('',(0.,0.,-1.)) ;
#32474=DIRECTION('',(0.,1.,0.)) ;
#32475=DIRECTION('center_axis',(0.,1.,0.)) ;
#32476=DIRECTION('ref_axis',(0.,0.,1.)) ;
#32477=DIRECTION('',(1.,0.,0.)) ;
#32478=DIRECTION('',(0.,0.,-1.)) ;
#32479=DIRECTION('',(-1.,0.,0.)) ;
#32480=DIRECTION('center_axis',(0.,0.,1.)) ;
#32481=DIRECTION('ref_axis',(1.,0.,0.)) ;
#32482=DIRECTION('',(-1.,0.,0.)) ;
#32483=DIRECTION('',(0.,-1.,0.)) ;
#32484=DIRECTION('',(1.,0.,0.)) ;
#32485=DIRECTION('center_axis',(0.,1.,0.)) ;
#32486=DIRECTION('ref_axis',(0.,0.,1.)) ;
#32487=DIRECTION('',(0.,0.,-1.)) ;
#32488=DIRECTION('',(-1.,0.,0.)) ;
#32489=DIRECTION('center_axis',(0.,0.,1.)) ;
#32490=DIRECTION('ref_axis',(1.,0.,0.)) ;
#32491=DIRECTION('',(0.,-1.,0.)) ;
#32492=DIRECTION('center_axis',(0.,0.,1.)) ;
#32493=DIRECTION('ref_axis',(1.,0.,0.)) ;
#32494=DIRECTION('',(0.,1.,0.)) ;
#32495=DIRECTION('',(1.,0.,0.)) ;
#32496=DIRECTION('center_axis',(1.,0.,0.)) ;
#32497=DIRECTION('ref_axis',(0.,0.,-1.)) ;
#32498=DIRECTION('',(0.,0.,-1.)) ;
#32499=DIRECTION('',(0.,-1.,0.)) ;
#32500=DIRECTION('center_axis',(0.,-1.,0.)) ;
#32501=DIRECTION('ref_axis',(0.,0.,-1.)) ;
#32502=DIRECTION('center_axis',(0.,0.,1.)) ;
#32503=DIRECTION('ref_axis',(0.707106781186547,-0.707106781186548,0.)) ;
#32504=DIRECTION('center_axis',(0.,0.,1.)) ;
#32505=DIRECTION('ref_axis',(1.,0.,0.)) ;
#32506=DIRECTION('',(0.707106781186547,-0.707106781186548,0.)) ;
#32507=DIRECTION('',(0.707106781186548,0.707106781186547,0.)) ;
#32508=DIRECTION('',(-0.707106781186547,0.707106781186548,0.)) ;
#32509=DIRECTION('center_axis',(0.707106781186548,0.707106781186547,0.)) ;
#32510=DIRECTION('ref_axis',(0.,0.,1.)) ;
#32511=DIRECTION('',(-0.707106781186547,0.707106781186548,0.)) ;
#32512=DIRECTION('',(0.,0.,-1.)) ;
#32513=DIRECTION('center_axis',(-0.707106781186548,-0.707106781186547,0.)) ;
#32514=DIRECTION('ref_axis',(0.,0.,-1.)) ;
#32515=DIRECTION('',(0.,0.,-1.)) ;
#32516=DIRECTION('',(0.707106781186547,-0.707106781186548,0.)) ;
#32517=DIRECTION('center_axis',(-0.707106781186548,-0.707106781186547,0.)) ;
#32518=DIRECTION('ref_axis',(0.,0.,-1.)) ;
#32519=DIRECTION('',(0.707106781186547,-0.707106781186548,0.)) ;
#32520=DIRECTION('',(0.,0.,-1.)) ;
#32521=DIRECTION('',(-0.707106781186547,0.707106781186548,0.)) ;
#32522=DIRECTION('center_axis',(0.,0.,1.)) ;
#32523=DIRECTION('ref_axis',(0.707106781186547,-0.707106781186548,0.)) ;
#32524=DIRECTION('center_axis',(0.,0.,-1.)) ;
#32525=DIRECTION('ref_axis',(1.,0.,0.)) ;
#32526=DIRECTION('',(-0.707106781186548,-0.707106781186547,0.)) ;
#32527=DIRECTION('center_axis',(0.,0.,1.)) ;
#32528=DIRECTION('ref_axis',(0.707106781186547,-0.707106781186548,0.)) ;
#32529=DIRECTION('center_axis',(0.,0.,1.)) ;
#32530=DIRECTION('ref_axis',(1.,0.,0.)) ;
#32531=DIRECTION('',(-0.707106781186547,0.707106781186548,0.)) ;
#32532=DIRECTION('',(0.707106781186548,0.707106781186547,0.)) ;
#32533=DIRECTION('center_axis',(0.,0.,1.)) ;
#32534=DIRECTION('ref_axis',(0.707106781186547,-0.707106781186548,0.)) ;
#32535=DIRECTION('center_axis',(0.,0.,-1.)) ;
#32536=DIRECTION('ref_axis',(1.,0.,0.)) ;
#32537=DIRECTION('',(-0.707106781186548,-0.707106781186547,0.)) ;
#32538=DIRECTION('',(0.707106781186547,-0.707106781186548,0.)) ;
#32539=DIRECTION('center_axis',(0.707106781186548,0.707106781186547,0.)) ;
#32540=DIRECTION('ref_axis',(0.,0.,1.)) ;
#32541=DIRECTION('',(0.,0.,-1.)) ;
#32542=DIRECTION('center_axis',(0.707106781186547,-0.707106781186548,0.)) ;
#32543=DIRECTION('ref_axis',(0.,0.,-1.)) ;
#32544=DIRECTION('center_axis',(-0.707106781186547,0.707106781186548,0.)) ;
#32545=DIRECTION('ref_axis',(0.,0.,1.)) ;
#32546=DIRECTION('center_axis',(0.,0.,1.)) ;
#32547=DIRECTION('ref_axis',(-0.707106781186548,-0.707106781186547,0.)) ;
#32548=DIRECTION('center_axis',(0.,0.,1.)) ;
#32549=DIRECTION('ref_axis',(1.,0.,0.)) ;
#32550=DIRECTION('',(-0.707106781186548,-0.707106781186547,0.)) ;
#32551=DIRECTION('',(0.707106781186547,-0.707106781186548,0.)) ;
#32552=DIRECTION('',(0.707106781186548,0.707106781186547,0.)) ;
#32553=DIRECTION('center_axis',(0.707106781186547,-0.707106781186548,0.)) ;
#32554=DIRECTION('ref_axis',(0.,0.,1.)) ;
#32555=DIRECTION('',(0.707106781186548,0.707106781186547,0.)) ;
#32556=DIRECTION('',(0.,0.,-1.)) ;
#32557=DIRECTION('center_axis',(-0.707106781186547,0.707106781186548,0.)) ;
#32558=DIRECTION('ref_axis',(0.,0.,-1.)) ;
#32559=DIRECTION('',(0.,0.,-1.)) ;
#32560=DIRECTION('',(-0.707106781186548,-0.707106781186547,0.)) ;
#32561=DIRECTION('center_axis',(-0.707106781186547,0.707106781186548,0.)) ;
#32562=DIRECTION('ref_axis',(0.,0.,-1.)) ;
#32563=DIRECTION('',(-0.707106781186548,-0.707106781186547,0.)) ;
#32564=DIRECTION('',(0.,0.,-1.)) ;
#32565=DIRECTION('',(0.707106781186548,0.707106781186547,0.)) ;
#32566=DIRECTION('center_axis',(0.,0.,1.)) ;
#32567=DIRECTION('ref_axis',(-0.707106781186548,-0.707106781186547,0.)) ;
#32568=DIRECTION('center_axis',(0.,0.,-1.)) ;
#32569=DIRECTION('ref_axis',(1.,0.,0.)) ;
#32570=DIRECTION('',(-0.707106781186547,0.707106781186548,0.)) ;
#32571=DIRECTION('center_axis',(0.,0.,1.)) ;
#32572=DIRECTION('ref_axis',(-0.707106781186548,-0.707106781186547,0.)) ;
#32573=DIRECTION('center_axis',(0.,0.,1.)) ;
#32574=DIRECTION('ref_axis',(1.,0.,0.)) ;
#32575=DIRECTION('',(0.707106781186548,0.707106781186547,0.)) ;
#32576=DIRECTION('',(0.707106781186547,-0.707106781186548,0.)) ;
#32577=DIRECTION('center_axis',(0.,0.,1.)) ;
#32578=DIRECTION('ref_axis',(-0.707106781186548,-0.707106781186547,0.)) ;
#32579=DIRECTION('center_axis',(0.,0.,-1.)) ;
#32580=DIRECTION('ref_axis',(1.,0.,0.)) ;
#32581=DIRECTION('',(-0.707106781186547,0.707106781186548,0.)) ;
#32582=DIRECTION('',(-0.707106781186548,-0.707106781186547,0.)) ;
#32583=DIRECTION('center_axis',(0.707106781186547,-0.707106781186548,0.)) ;
#32584=DIRECTION('ref_axis',(0.,0.,1.)) ;
#32585=DIRECTION('',(0.,0.,-1.)) ;
#32586=DIRECTION('center_axis',(-0.707106781186548,-0.707106781186547,0.)) ;
#32587=DIRECTION('ref_axis',(0.,0.,-1.)) ;
#32588=DIRECTION('center_axis',(0.707106781186548,0.707106781186547,0.)) ;
#32589=DIRECTION('ref_axis',(0.,0.,1.)) ;
#32590=DIRECTION('center_axis',(0.,0.,1.)) ;
#32591=DIRECTION('ref_axis',(-0.707106781186547,0.707106781186548,0.)) ;
#32592=DIRECTION('center_axis',(0.,0.,1.)) ;
#32593=DIRECTION('ref_axis',(1.,0.,0.)) ;
#32594=DIRECTION('',(-0.707106781186547,0.707106781186548,0.)) ;
#32595=DIRECTION('',(-0.707106781186548,-0.707106781186547,0.)) ;
#32596=DIRECTION('',(0.707106781186547,-0.707106781186548,0.)) ;
#32597=DIRECTION('center_axis',(-0.707106781186548,-0.707106781186547,0.)) ;
#32598=DIRECTION('ref_axis',(0.,0.,1.)) ;
#32599=DIRECTION('',(0.707106781186547,-0.707106781186548,0.)) ;
#32600=DIRECTION('',(0.,0.,-1.)) ;
#32601=DIRECTION('center_axis',(0.707106781186548,0.707106781186547,0.)) ;
#32602=DIRECTION('ref_axis',(0.,0.,-1.)) ;
#32603=DIRECTION('',(0.,0.,-1.)) ;
#32604=DIRECTION('',(-0.707106781186547,0.707106781186548,0.)) ;
#32605=DIRECTION('center_axis',(0.707106781186548,0.707106781186547,0.)) ;
#32606=DIRECTION('ref_axis',(0.,0.,-1.)) ;
#32607=DIRECTION('',(-0.707106781186547,0.707106781186548,0.)) ;
#32608=DIRECTION('',(0.,0.,-1.)) ;
#32609=DIRECTION('',(0.707106781186547,-0.707106781186548,0.)) ;
#32610=DIRECTION('center_axis',(0.,0.,1.)) ;
#32611=DIRECTION('ref_axis',(-0.707106781186547,0.707106781186548,0.)) ;
#32612=DIRECTION('center_axis',(0.,0.,-1.)) ;
#32613=DIRECTION('ref_axis',(1.,0.,0.)) ;
#32614=DIRECTION('',(0.707106781186548,0.707106781186547,0.)) ;
#32615=DIRECTION('center_axis',(0.,0.,1.)) ;
#32616=DIRECTION('ref_axis',(-0.707106781186547,0.707106781186548,0.)) ;
#32617=DIRECTION('center_axis',(0.,0.,1.)) ;
#32618=DIRECTION('ref_axis',(1.,0.,0.)) ;
#32619=DIRECTION('',(0.707106781186547,-0.707106781186548,0.)) ;
#32620=DIRECTION('',(-0.707106781186548,-0.707106781186547,0.)) ;
#32621=DIRECTION('center_axis',(0.,0.,1.)) ;
#32622=DIRECTION('ref_axis',(-0.707106781186547,0.707106781186548,0.)) ;
#32623=DIRECTION('center_axis',(0.,0.,-1.)) ;
#32624=DIRECTION('ref_axis',(1.,0.,0.)) ;
#32625=DIRECTION('',(0.707106781186548,0.707106781186547,0.)) ;
#32626=DIRECTION('',(-0.707106781186547,0.707106781186548,0.)) ;
#32627=DIRECTION('center_axis',(-0.707106781186548,-0.707106781186547,0.)) ;
#32628=DIRECTION('ref_axis',(0.,0.,1.)) ;
#32629=DIRECTION('',(0.,0.,-1.)) ;
#32630=DIRECTION('center_axis',(-0.707106781186547,0.707106781186548,0.)) ;
#32631=DIRECTION('ref_axis',(0.,0.,-1.)) ;
#32632=DIRECTION('center_axis',(0.707106781186547,-0.707106781186548,0.)) ;
#32633=DIRECTION('ref_axis',(0.,0.,1.)) ;
#32634=DIRECTION('center_axis',(0.,0.,1.)) ;
#32635=DIRECTION('ref_axis',(0.707106781186548,0.707106781186547,0.)) ;
#32636=DIRECTION('center_axis',(0.,0.,1.)) ;
#32637=DIRECTION('ref_axis',(1.,0.,0.)) ;
#32638=DIRECTION('',(0.707106781186548,0.707106781186547,0.)) ;
#32639=DIRECTION('',(-0.707106781186547,0.707106781186548,0.)) ;
#32640=DIRECTION('',(-0.707106781186548,-0.707106781186547,0.)) ;
#32641=DIRECTION('center_axis',(-0.707106781186547,0.707106781186548,0.)) ;
#32642=DIRECTION('ref_axis',(0.,0.,1.)) ;
#32643=DIRECTION('',(-0.707106781186548,-0.707106781186547,0.)) ;
#32644=DIRECTION('',(0.,0.,-1.)) ;
#32645=DIRECTION('center_axis',(0.707106781186547,-0.707106781186548,0.)) ;
#32646=DIRECTION('ref_axis',(0.,0.,-1.)) ;
#32647=DIRECTION('',(0.,0.,-1.)) ;
#32648=DIRECTION('',(0.707106781186548,0.707106781186547,0.)) ;
#32649=DIRECTION('center_axis',(0.707106781186547,-0.707106781186548,0.)) ;
#32650=DIRECTION('ref_axis',(0.,0.,-1.)) ;
#32651=DIRECTION('',(0.707106781186548,0.707106781186547,0.)) ;
#32652=DIRECTION('',(0.,0.,-1.)) ;
#32653=DIRECTION('',(-0.707106781186548,-0.707106781186547,0.)) ;
#32654=DIRECTION('center_axis',(0.,0.,1.)) ;
#32655=DIRECTION('ref_axis',(0.707106781186548,0.707106781186547,0.)) ;
#32656=DIRECTION('center_axis',(0.,0.,-1.)) ;
#32657=DIRECTION('ref_axis',(1.,0.,0.)) ;
#32658=DIRECTION('',(0.707106781186547,-0.707106781186548,0.)) ;
#32659=DIRECTION('center_axis',(0.,0.,1.)) ;
#32660=DIRECTION('ref_axis',(0.707106781186548,0.707106781186547,0.)) ;
#32661=DIRECTION('center_axis',(0.,0.,1.)) ;
#32662=DIRECTION('ref_axis',(1.,0.,0.)) ;
#32663=DIRECTION('',(-0.707106781186548,-0.707106781186547,0.)) ;
#32664=DIRECTION('',(-0.707106781186547,0.707106781186548,0.)) ;
#32665=DIRECTION('center_axis',(0.,0.,1.)) ;
#32666=DIRECTION('ref_axis',(0.707106781186548,0.707106781186547,0.)) ;
#32667=DIRECTION('center_axis',(0.,0.,-1.)) ;
#32668=DIRECTION('ref_axis',(1.,0.,0.)) ;
#32669=DIRECTION('',(0.707106781186547,-0.707106781186548,0.)) ;
#32670=DIRECTION('',(0.707106781186548,0.707106781186547,0.)) ;
#32671=DIRECTION('center_axis',(-0.707106781186547,0.707106781186548,0.)) ;
#32672=DIRECTION('ref_axis',(0.,0.,1.)) ;
#32673=DIRECTION('',(0.,0.,-1.)) ;
#32674=DIRECTION('center_axis',(0.707106781186548,0.707106781186547,0.)) ;
#32675=DIRECTION('ref_axis',(0.,0.,-1.)) ;
#32676=DIRECTION('center_axis',(-0.707106781186548,-0.707106781186547,0.)) ;
#32677=DIRECTION('ref_axis',(0.,0.,1.)) ;
#32678=DIRECTION('center_axis',(0.,0.,1.)) ;
#32679=DIRECTION('ref_axis',(1.,0.,0.)) ;
#32680=DIRECTION('center_axis',(0.,0.,1.)) ;
#32681=DIRECTION('ref_axis',(1.,0.,0.)) ;
#32682=DIRECTION('',(0.,0.,1.)) ;
#32683=DIRECTION('center_axis',(0.,0.,-1.)) ;
#32684=DIRECTION('ref_axis',(1.,0.,0.)) ;
#32685=DIRECTION('center_axis',(0.,0.,1.)) ;
#32686=DIRECTION('ref_axis',(1.,0.,0.)) ;
#32687=DIRECTION('center_axis',(0.,0.,-1.)) ;
#32688=DIRECTION('ref_axis',(1.,0.,0.)) ;
#32689=DIRECTION('',(0.,0.,1.)) ;
#32690=DIRECTION('center_axis',(0.,0.,-1.)) ;
#32691=DIRECTION('ref_axis',(1.,0.,0.)) ;
#32692=DIRECTION('center_axis',(0.,0.,-1.)) ;
#32693=DIRECTION('ref_axis',(-1.,0.,0.)) ;
#32694=DIRECTION('center_axis',(0.,0.,1.)) ;
#32695=DIRECTION('ref_axis',(1.,0.,0.)) ;
#32696=DIRECTION('center_axis',(0.,0.,1.)) ;
#32697=DIRECTION('ref_axis',(1.,0.,0.)) ;
#32698=DIRECTION('center_axis',(0.,0.,1.)) ;
#32699=DIRECTION('ref_axis',(1.,0.,0.)) ;
#32700=DIRECTION('',(-0.565399080761227,-6.92414174495092E-17,0.824817482522261)) ;
#32701=DIRECTION('center_axis',(0.,0.,1.)) ;
#32702=DIRECTION('ref_axis',(1.,0.,0.)) ;
#32703=DIRECTION('',(0.565399080761227,6.92414174495092E-17,-0.824817482522261)) ;
#32704=DIRECTION('center_axis',(0.,0.,-1.)) ;
#32705=DIRECTION('ref_axis',(1.,0.,0.)) ;
#32706=DIRECTION('center_axis',(0.,0.,-1.)) ;
#32707=DIRECTION('ref_axis',(-1.,0.,0.)) ;
#41225=CARTESIAN_POINT('',(0.,0.,0.)) ;
#41226=CARTESIAN_POINT('Origin',(-4.9,56.8,112.3)) ;
#41227=CARTESIAN_POINT('',(-4.2,56.8,111.68)) ;
#41228=CARTESIAN_POINT('Origin',(-4.2,56.8,112.3)) ;
#41229=CARTESIAN_POINT('',(-5.6,56.8,111.68)) ;
#41230=CARTESIAN_POINT('',(-4.9,56.8,111.68)) ;
#41231=CARTESIAN_POINT('Origin',(-5.6,56.8,112.3)) ;
#41232=CARTESIAN_POINT('Origin',(-4.2,56.25,108.5)) ;
#41233=CARTESIAN_POINT('',(-4.2,54.8394018931644,109.)) ;
#41234=CARTESIAN_POINT('',(-4.2,54.8394018931644,110.)) ;
#41235=CARTESIAN_POINT('',(-4.2,54.8394018931644,110.)) ;
#41236=CARTESIAN_POINT('',(-4.2,54.5,109.)) ;
#41237=CARTESIAN_POINT('',(-4.2,28.125,109.)) ;
#41238=CARTESIAN_POINT('',(-4.2,54.5,107.)) ;
#41239=CARTESIAN_POINT('',(-4.2,54.5,108.5)) ;
#41240=CARTESIAN_POINT('',(-4.2,58.,107.)) ;
#41241=CARTESIAN_POINT('',(-4.2,56.25,107.)) ;
#41242=CARTESIAN_POINT('',(-4.2,58.,113.2)) ;
#41243=CARTESIAN_POINT('',(-4.2,58.,111.6)) ;
#41244=CARTESIAN_POINT('',(-4.2,55.6,113.2)) ;
#41245=CARTESIAN_POINT('',(-4.2,56.8,113.2)) ;
#41246=CARTESIAN_POINT('',(-4.2,55.6,110.)) ;
#41247=CARTESIAN_POINT('',(-4.2,55.6,111.6)) ;
#41248=CARTESIAN_POINT('',(-4.2,56.25,110.)) ;
#41249=CARTESIAN_POINT('Origin',(-4.9,54.5,108.5)) ;
#41250=CARTESIAN_POINT('',(-5.6,54.5,109.)) ;
#41251=CARTESIAN_POINT('',(-2.45,54.5,109.)) ;
#41252=CARTESIAN_POINT('',(-5.6,54.5,107.)) ;
#41253=CARTESIAN_POINT('',(-5.6,54.5,108.5)) ;
#41254=CARTESIAN_POINT('',(-4.9,54.5,107.)) ;
#41255=CARTESIAN_POINT('Origin',(-4.9,56.8,113.2)) ;
#41256=CARTESIAN_POINT('',(-5.6,58.,113.2)) ;
#41257=CARTESIAN_POINT('',(-4.9,58.,113.2)) ;
#41258=CARTESIAN_POINT('',(-5.6,55.6,113.2)) ;
#41259=CARTESIAN_POINT('',(-5.6,56.8,113.2)) ;
#41260=CARTESIAN_POINT('',(-4.9,55.6,113.2)) ;
#41261=CARTESIAN_POINT('Origin',(-4.9,55.6,111.6)) ;
#41262=CARTESIAN_POINT('',(-5.6,55.6,110.)) ;
#41263=CARTESIAN_POINT('',(-5.6,55.6,111.6)) ;
#41264=CARTESIAN_POINT('',(-4.9,55.6,110.)) ;
#41265=CARTESIAN_POINT('Origin',(-4.9,56.25,110.)) ;
#41266=CARTESIAN_POINT('',(-5.6,54.7141663557072,110.)) ;
#41267=CARTESIAN_POINT('Origin',(0.,0.,110.)) ;
#41268=CARTESIAN_POINT('',(-5.6,56.25,110.)) ;
#41269=CARTESIAN_POINT('Origin',(-4.9,56.25,107.)) ;
#41270=CARTESIAN_POINT('',(-5.6,58.,107.)) ;
#41271=CARTESIAN_POINT('',(-5.6,56.25,107.)) ;
#41272=CARTESIAN_POINT('',(-4.9,58.,107.)) ;
#41273=CARTESIAN_POINT('Origin',(-5.6,56.25,108.5)) ;
#41274=CARTESIAN_POINT('',(-5.6,54.7141663557072,109.)) ;
#41275=CARTESIAN_POINT('',(-5.6,54.7141663557072,110.)) ;
#41276=CARTESIAN_POINT('',(-5.6,58.,111.6)) ;
#41277=CARTESIAN_POINT('',(-5.6,28.125,109.)) ;
#41278=CARTESIAN_POINT('Origin',(-4.9,58.,108.5)) ;
#41279=CARTESIAN_POINT('Origin',(0.,0.,110.)) ;
#41280=CARTESIAN_POINT('',(-55.,-6.73555739531044E-15,111.)) ;
#41281=CARTESIAN_POINT('Origin',(0.,0.,111.)) ;
#41282=CARTESIAN_POINT('',(-55.,-6.73555739531044E-15,109.)) ;
#41283=CARTESIAN_POINT('',(-55.,-6.73555739531044E-15,110.)) ;
#41284=CARTESIAN_POINT('',(5.6,54.7141663557072,109.)) ;
#41285=CARTESIAN_POINT('Origin',(0.,0.,109.)) ;
#41286=CARTESIAN_POINT('',(5.6,54.7141663557072,110.)) ;
#41287=CARTESIAN_POINT('',(5.6,54.7141663557072,110.)) ;
#41288=CARTESIAN_POINT('',(4.2,54.8394018931644,110.)) ;
#41289=CARTESIAN_POINT('Origin',(0.,0.,110.)) ;
#41290=CARTESIAN_POINT('',(4.2,54.8394018931644,109.)) ;
#41291=CARTESIAN_POINT('',(4.2,54.8394018931644,110.)) ;
#41292=CARTESIAN_POINT('Origin',(0.,0.,109.)) ;
#41293=CARTESIAN_POINT('Origin',(0.,0.,109.)) ;
#41294=CARTESIAN_POINT('Origin',(4.9,56.8,112.3)) ;
#41295=CARTESIAN_POINT('',(4.2,56.8,112.92)) ;
#41296=CARTESIAN_POINT('Origin',(4.2,56.8,112.3)) ;
#41297=CARTESIAN_POINT('',(5.6,56.8,112.92)) ;
#41298=CARTESIAN_POINT('',(4.9,56.8,112.92)) ;
#41299=CARTESIAN_POINT('Origin',(5.6,56.8,112.3)) ;
#41300=CARTESIAN_POINT('Origin',(5.6,56.25,108.5)) ;
#41301=CARTESIAN_POINT('',(5.6,54.5,109.)) ;
#41302=CARTESIAN_POINT('',(5.6,28.125,109.)) ;
#41303=CARTESIAN_POINT('',(5.6,54.5,107.)) ;
#41304=CARTESIAN_POINT('',(5.6,54.5,108.5)) ;
#41305=CARTESIAN_POINT('',(5.6,58.,107.)) ;
#41306=CARTESIAN_POINT('',(5.6,56.25,107.)) ;
#41307=CARTESIAN_POINT('',(5.6,58.,113.2)) ;
#41308=CARTESIAN_POINT('',(5.6,58.,111.6)) ;
#41309=CARTESIAN_POINT('',(5.6,55.6,113.2)) ;
#41310=CARTESIAN_POINT('',(5.6,56.8,113.2)) ;
#41311=CARTESIAN_POINT('',(5.6,55.6,110.)) ;
#41312=CARTESIAN_POINT('',(5.6,55.6,111.6)) ;
#41313=CARTESIAN_POINT('',(5.6,56.25,110.)) ;
#41314=CARTESIAN_POINT('Origin',(4.9,54.5,108.5)) ;
#41315=CARTESIAN_POINT('',(4.2,54.5,109.)) ;
#41316=CARTESIAN_POINT('',(2.45,54.5,109.)) ;
#41317=CARTESIAN_POINT('',(4.2,54.5,107.)) ;
#41318=CARTESIAN_POINT('',(4.2,54.5,108.5)) ;
#41319=CARTESIAN_POINT('',(4.9,54.5,107.)) ;
#41320=CARTESIAN_POINT('Origin',(4.9,56.8,113.2)) ;
#41321=CARTESIAN_POINT('',(4.2,58.,113.2)) ;
#41322=CARTESIAN_POINT('',(4.9,58.,113.2)) ;
#41323=CARTESIAN_POINT('',(4.2,55.6,113.2)) ;
#41324=CARTESIAN_POINT('',(4.2,56.8,113.2)) ;
#41325=CARTESIAN_POINT('',(4.9,55.6,113.2)) ;
#41326=CARTESIAN_POINT('Origin',(4.9,55.6,111.6)) ;
#41327=CARTESIAN_POINT('',(4.2,55.6,110.)) ;
#41328=CARTESIAN_POINT('',(4.2,55.6,111.6)) ;
#41329=CARTESIAN_POINT('',(4.9,55.6,110.)) ;
#41330=CARTESIAN_POINT('Origin',(4.9,56.25,110.)) ;
#41331=CARTESIAN_POINT('',(4.2,56.25,110.)) ;
#41332=CARTESIAN_POINT('Origin',(4.9,56.25,107.)) ;
#41333=CARTESIAN_POINT('',(4.2,58.,107.)) ;
#41334=CARTESIAN_POINT('',(4.2,56.25,107.)) ;
#41335=CARTESIAN_POINT('',(4.9,58.,107.)) ;
#41336=CARTESIAN_POINT('Origin',(4.2,56.25,108.5)) ;
#41337=CARTESIAN_POINT('',(4.2,58.,111.6)) ;
#41338=CARTESIAN_POINT('',(4.2,28.125,109.)) ;
#41339=CARTESIAN_POINT('Origin',(4.9,58.,108.5)) ;
#41340=CARTESIAN_POINT('Origin',(20.7889393668845,-20.7889393668845,73.2)) ;
#41341=CARTESIAN_POINT('',(18.5017201441464,-22.0372540500791,73.2)) ;
#41342=CARTESIAN_POINT('',(22.0372540500791,-18.5017201441464,73.2)) ;
#41343=CARTESIAN_POINT('Origin',(0.,0.,73.2)) ;
#41344=CARTESIAN_POINT('',(20.8596500450031,-24.3951839509359,73.2)) ;
#41345=CARTESIAN_POINT('',(19.0211724139181,-22.5567063198509,73.2)) ;
#41346=CARTESIAN_POINT('',(24.3951839509359,-20.8596500450032,73.2)) ;
#41347=CARTESIAN_POINT('',(22.6274169979695,-22.6274169979695,73.2)) ;
#41348=CARTESIAN_POINT('',(22.5567063198509,-19.0211724139181,73.2)) ;
#41349=CARTESIAN_POINT('Origin',(19.0211724139181,-22.5567063198509,72.6)) ;
#41350=CARTESIAN_POINT('',(17.9177945565738,-21.4533284625066,72.)) ;
#41351=CARTESIAN_POINT('Ctrl Pts',(17.9177945565738,-21.4533284625066,72.)) ;
#41352=CARTESIAN_POINT('Ctrl Pts',(18.2055235988788,-21.7410575048115,72.5912312611487)) ;
#41353=CARTESIAN_POINT('Ctrl Pts',(18.5017201441464,-22.0372540500791,73.2)) ;
#41354=CARTESIAN_POINT('',(20.8596500450031,-24.3951839509359,72.)) ;
#41355=CARTESIAN_POINT('',(19.0211724139181,-22.5567063198509,72.)) ;
#41356=CARTESIAN_POINT('',(20.8596500450031,-24.3951839509359,72.6)) ;
#41357=CARTESIAN_POINT('Origin',(22.5567063198509,-19.0211724139181,72.6)) ;
#41358=CARTESIAN_POINT('',(21.4533284625065,-17.9177945565738,72.)) ;
#41359=CARTESIAN_POINT('Ctrl Pts',(22.0372540500791,-18.5017201441464,73.2)) ;
#41360=CARTESIAN_POINT('Ctrl Pts',(21.7410575071122,-18.2055236011795,72.5912312658768)) ;
#41361=CARTESIAN_POINT('Ctrl Pts',(21.4533284625065,-17.9177945565738,72.)) ;
#41362=CARTESIAN_POINT('',(24.3951839509359,-20.8596500450032,72.)) ;
#41363=CARTESIAN_POINT('',(24.3951839509359,-20.8596500450032,72.6)) ;
#41364=CARTESIAN_POINT('',(22.5567063198509,-19.0211724139181,72.)) ;
#41365=CARTESIAN_POINT('Origin',(22.5567063198509,-19.0211724139181,72.6)) ;
#41366=CARTESIAN_POINT('',(21.0273194971963,-17.4917855912636,72.)) ;
#41367=CARTESIAN_POINT('',(21.6113450338214,-18.0758111278886,73.2)) ;
#41368=CARTESIAN_POINT('Ctrl Pts',(21.0273194971963,-17.4917855912636,72.)) ;
#41369=CARTESIAN_POINT('Ctrl Pts',(21.3150062821372,-17.7794723762045,72.5910387012431)) ;
#41370=CARTESIAN_POINT('Ctrl Pts',(21.6113450338214,-18.0758111278886,73.2)) ;
#41371=CARTESIAN_POINT('',(20.7182286887658,-17.1826947828331,72.)) ;
#41372=CARTESIAN_POINT('',(22.5567063198509,-19.0211724139181,72.)) ;
#41373=CARTESIAN_POINT('',(20.7182286887658,-17.1826947828331,73.2)) ;
#41374=CARTESIAN_POINT('',(20.7182286887658,-17.1826947828331,72.6)) ;
#41375=CARTESIAN_POINT('',(22.5567063198509,-19.0211724139181,73.2)) ;
#41376=CARTESIAN_POINT('Origin',(20.7889393668845,-20.7889393668845,72.)) ;
#41377=CARTESIAN_POINT('Origin',(0.,0.,72.)) ;
#41378=CARTESIAN_POINT('',(22.6274169979695,-22.6274169979695,72.)) ;
#41379=CARTESIAN_POINT('Origin',(20.7889393668845,-20.7889393668845,72.)) ;
#41380=CARTESIAN_POINT('',(17.4917855912636,-21.0273194971963,72.)) ;
#41381=CARTESIAN_POINT('Origin',(0.,0.,72.)) ;
#41382=CARTESIAN_POINT('',(17.1826947828331,-20.7182286887659,72.)) ;
#41383=CARTESIAN_POINT('',(19.0211724139181,-22.5567063198509,72.)) ;
#41384=CARTESIAN_POINT('',(18.9504617357995,-18.9504617357995,72.)) ;
#41385=CARTESIAN_POINT('Origin',(20.7889393668845,-20.7889393668845,73.2)) ;
#41386=CARTESIAN_POINT('',(18.0758111278886,-21.6113450338214,73.2)) ;
#41387=CARTESIAN_POINT('Origin',(0.,0.,73.2)) ;
#41388=CARTESIAN_POINT('',(17.1826947828331,-20.7182286887659,73.2)) ;
#41389=CARTESIAN_POINT('',(18.9504617357995,-18.9504617357995,73.2)) ;
#41390=CARTESIAN_POINT('',(19.0211724139181,-22.5567063198509,73.2)) ;
#41391=CARTESIAN_POINT('Origin',(19.0211724139181,-22.5567063198509,72.6)) ;
#41392=CARTESIAN_POINT('Ctrl Pts',(18.0758111278886,-21.6113450338214,73.2)) ;
#41393=CARTESIAN_POINT('Ctrl Pts',(17.7794723670287,-21.3150062729614,72.5910386823896)) ;
#41394=CARTESIAN_POINT('Ctrl Pts',(17.4917855912636,-21.0273194971963,72.)) ;
#41395=CARTESIAN_POINT('',(17.1826947828331,-20.7182286887659,72.6)) ;
#41396=CARTESIAN_POINT('Origin',(18.9504617357995,-18.9504617357995,72.6)) ;
#41397=CARTESIAN_POINT('Origin',(22.6274169979695,-22.6274169979695,72.6)) ;
#41398=CARTESIAN_POINT('Origin',(-20.7889393668845,-20.7889393668845,73.2)) ;
#41399=CARTESIAN_POINT('',(-22.0372540500791,-18.5017201441464,73.2)) ;
#41400=CARTESIAN_POINT('',(-18.5017201441464,-22.0372540500791,73.2)) ;
#41401=CARTESIAN_POINT('Origin',(0.,0.,73.2)) ;
#41402=CARTESIAN_POINT('',(-24.3951839509359,-20.8596500450031,73.2)) ;
#41403=CARTESIAN_POINT('',(-22.5567063198509,-19.0211724139181,73.2)) ;
#41404=CARTESIAN_POINT('',(-20.8596500450032,-24.3951839509359,73.2)) ;
#41405=CARTESIAN_POINT('',(-22.6274169979695,-22.6274169979695,73.2)) ;
#41406=CARTESIAN_POINT('',(-19.0211724139181,-22.5567063198509,73.2)) ;
#41407=CARTESIAN_POINT('Origin',(-22.5567063198509,-19.0211724139181,72.6)) ;
#41408=CARTESIAN_POINT('',(-21.4533284625066,-17.9177945565738,72.)) ;
#41409=CARTESIAN_POINT('Ctrl Pts',(-21.4533284625066,-17.9177945565738,
72.)) ;
#41410=CARTESIAN_POINT('Ctrl Pts',(-21.7410575024954,-18.2055235965626,
72.591231256389)) ;
#41411=CARTESIAN_POINT('Ctrl Pts',(-22.0372540500791,-18.5017201441464,
73.2)) ;
#41412=CARTESIAN_POINT('',(-24.3951839509359,-20.8596500450031,72.)) ;
#41413=CARTESIAN_POINT('',(-22.5567063198509,-19.0211724139181,72.)) ;
#41414=CARTESIAN_POINT('',(-24.3951839509359,-20.8596500450031,72.6)) ;
#41415=CARTESIAN_POINT('Origin',(-19.0211724139181,-22.5567063198509,72.6)) ;
#41416=CARTESIAN_POINT('',(-17.9177945565738,-21.4533284625065,72.)) ;
#41417=CARTESIAN_POINT('Ctrl Pts',(-18.5017201441464,-22.0372540500791,
73.2)) ;
#41418=CARTESIAN_POINT('Ctrl Pts',(-18.2055235965626,-21.7410575024954,
72.591231256389)) ;
#41419=CARTESIAN_POINT('Ctrl Pts',(-17.9177945565738,-21.4533284625066,
72.)) ;
#41420=CARTESIAN_POINT('',(-20.8596500450032,-24.3951839509359,72.)) ;
#41421=CARTESIAN_POINT('',(-20.8596500450032,-24.3951839509359,72.6)) ;
#41422=CARTESIAN_POINT('',(-19.0211724139181,-22.5567063198509,72.)) ;
#41423=CARTESIAN_POINT('Origin',(-19.0211724139181,-22.5567063198509,72.6)) ;
#41424=CARTESIAN_POINT('',(-17.4917855912636,-21.0273194971963,72.)) ;
#41425=CARTESIAN_POINT('',(-18.0758111278886,-21.6113450338214,73.2)) ;
#41426=CARTESIAN_POINT('Ctrl Pts',(-17.4917855912636,-21.0273194971963,
72.)) ;
#41427=CARTESIAN_POINT('Ctrl Pts',(-17.7794723741827,-21.3150062801154,
72.5910386970889)) ;
#41428=CARTESIAN_POINT('Ctrl Pts',(-18.0758111278886,-21.6113450338214,
73.2)) ;
#41429=CARTESIAN_POINT('',(-17.1826947828331,-20.7182286887658,72.)) ;
#41430=CARTESIAN_POINT('',(-19.0211724139181,-22.5567063198509,72.)) ;
#41431=CARTESIAN_POINT('',(-17.1826947828331,-20.7182286887658,73.2)) ;
#41432=CARTESIAN_POINT('',(-17.1826947828331,-20.7182286887658,72.6)) ;
#41433=CARTESIAN_POINT('',(-19.0211724139181,-22.5567063198509,73.2)) ;
#41434=CARTESIAN_POINT('Origin',(-20.7889393668845,-20.7889393668845,72.)) ;
#41435=CARTESIAN_POINT('Origin',(0.,0.,72.)) ;
#41436=CARTESIAN_POINT('',(-22.6274169979695,-22.6274169979695,72.)) ;
#41437=CARTESIAN_POINT('Origin',(-20.7889393668845,-20.7889393668845,72.)) ;
#41438=CARTESIAN_POINT('',(-21.0273194971963,-17.4917855912636,72.)) ;
#41439=CARTESIAN_POINT('Origin',(0.,0.,72.)) ;
#41440=CARTESIAN_POINT('',(-20.7182286887659,-17.1826947828331,72.)) ;
#41441=CARTESIAN_POINT('',(-22.5567063198509,-19.0211724139181,72.)) ;
#41442=CARTESIAN_POINT('',(-18.9504617357995,-18.9504617357995,72.)) ;
#41443=CARTESIAN_POINT('Origin',(-20.7889393668845,-20.7889393668845,73.2)) ;
#41444=CARTESIAN_POINT('',(-21.6113450338214,-18.0758111278886,73.2)) ;
#41445=CARTESIAN_POINT('Origin',(0.,0.,73.2)) ;
#41446=CARTESIAN_POINT('',(-20.7182286887659,-17.1826947828331,73.2)) ;
#41447=CARTESIAN_POINT('',(-18.9504617357995,-18.9504617357995,73.2)) ;
#41448=CARTESIAN_POINT('',(-22.5567063198509,-19.0211724139181,73.2)) ;
#41449=CARTESIAN_POINT('Origin',(-22.5567063198509,-19.0211724139181,72.6)) ;
#41450=CARTESIAN_POINT('Ctrl Pts',(-21.6113450338214,-18.0758111278886,
73.2)) ;
#41451=CARTESIAN_POINT('Ctrl Pts',(-21.3150062739694,-17.7794723680366,
72.5910386844606)) ;
#41452=CARTESIAN_POINT('Ctrl Pts',(-21.0273194971963,-17.4917855912636,
72.)) ;
#41453=CARTESIAN_POINT('',(-20.7182286887659,-17.1826947828331,72.6)) ;
#41454=CARTESIAN_POINT('Origin',(-18.9504617357995,-18.9504617357995,72.6)) ;
#41455=CARTESIAN_POINT('Origin',(-22.6274169979695,-22.6274169979695,72.6)) ;
#41456=CARTESIAN_POINT('Origin',(-20.7889393668845,20.7889393668845,73.2)) ;
#41457=CARTESIAN_POINT('',(-18.5017201441464,22.0372540500791,73.2)) ;
#41458=CARTESIAN_POINT('',(-22.0372540500791,18.5017201441464,73.2)) ;
#41459=CARTESIAN_POINT('Origin',(0.,0.,73.2)) ;
#41460=CARTESIAN_POINT('',(-20.8596500450031,24.3951839509359,73.2)) ;
#41461=CARTESIAN_POINT('',(-19.0211724139181,22.5567063198509,73.2)) ;
#41462=CARTESIAN_POINT('',(-24.3951839509359,20.8596500450032,73.2)) ;
#41463=CARTESIAN_POINT('',(-22.6274169979695,22.6274169979695,73.2)) ;
#41464=CARTESIAN_POINT('',(-22.5567063198509,19.0211724139181,73.2)) ;
#41465=CARTESIAN_POINT('Origin',(-19.0211724139181,22.5567063198509,72.6)) ;
#41466=CARTESIAN_POINT('',(-17.9177945565738,21.4533284625066,72.)) ;
#41467=CARTESIAN_POINT('Ctrl Pts',(-17.9177945565738,21.4533284625066,72.)) ;
#41468=CARTESIAN_POINT('Ctrl Pts',(-18.2055235965626,21.7410575024954,72.591231256389)) ;
#41469=CARTESIAN_POINT('Ctrl Pts',(-18.5017201441464,22.0372540500791,73.2)) ;
#41470=CARTESIAN_POINT('',(-20.8596500450031,24.3951839509359,72.)) ;
#41471=CARTESIAN_POINT('',(-19.0211724139181,22.5567063198509,72.)) ;
#41472=CARTESIAN_POINT('',(-20.8596500450031,24.3951839509359,72.6)) ;
#41473=CARTESIAN_POINT('Origin',(-22.5567063198509,19.0211724139181,72.6)) ;
#41474=CARTESIAN_POINT('',(-21.4533284625066,17.9177945565738,72.)) ;
#41475=CARTESIAN_POINT('Ctrl Pts',(-22.0372540500791,18.5017201441464,73.2)) ;
#41476=CARTESIAN_POINT('Ctrl Pts',(-21.7410575025031,18.2055235965704,72.5912312564048)) ;
#41477=CARTESIAN_POINT('Ctrl Pts',(-21.4533284625066,17.9177945565738,72.)) ;
#41478=CARTESIAN_POINT('',(-24.3951839509359,20.8596500450032,72.)) ;
#41479=CARTESIAN_POINT('',(-24.3951839509359,20.8596500450032,72.6)) ;
#41480=CARTESIAN_POINT('',(-22.5567063198509,19.0211724139181,72.)) ;
#41481=CARTESIAN_POINT('Origin',(-22.5567063198509,19.0211724139181,72.6)) ;
#41482=CARTESIAN_POINT('',(-21.0273194971963,17.4917855912636,72.)) ;
#41483=CARTESIAN_POINT('',(-21.6113450338214,18.0758111278886,73.2)) ;
#41484=CARTESIAN_POINT('Ctrl Pts',(-21.0273194971963,17.4917855912636,72.)) ;
#41485=CARTESIAN_POINT('Ctrl Pts',(-21.315006276006,17.7794723700733,72.5910386886453)) ;
#41486=CARTESIAN_POINT('Ctrl Pts',(-21.6113450338214,18.0758111278886,73.2)) ;
#41487=CARTESIAN_POINT('',(-20.7182286887658,17.1826947828331,72.)) ;
#41488=CARTESIAN_POINT('',(-22.5567063198509,19.0211724139181,72.)) ;
#41489=CARTESIAN_POINT('',(-20.7182286887658,17.1826947828331,73.2)) ;
#41490=CARTESIAN_POINT('',(-20.7182286887658,17.1826947828331,72.6)) ;
#41491=CARTESIAN_POINT('',(-22.5567063198509,19.0211724139181,73.2)) ;
#41492=CARTESIAN_POINT('Origin',(-20.7889393668845,20.7889393668845,72.)) ;
#41493=CARTESIAN_POINT('Origin',(0.,0.,72.)) ;
#41494=CARTESIAN_POINT('',(-22.6274169979695,22.6274169979695,72.)) ;
#41495=CARTESIAN_POINT('Origin',(-20.7889393668845,20.7889393668845,72.)) ;
#41496=CARTESIAN_POINT('',(-17.4917855912636,21.0273194971963,72.)) ;
#41497=CARTESIAN_POINT('Origin',(0.,0.,72.)) ;
#41498=CARTESIAN_POINT('',(-17.1826947828331,20.7182286887658,72.)) ;
#41499=CARTESIAN_POINT('',(-19.0211724139181,22.5567063198509,72.)) ;
#41500=CARTESIAN_POINT('',(-18.9504617357995,18.9504617357995,72.)) ;
#41501=CARTESIAN_POINT('Origin',(-20.7889393668845,20.7889393668845,73.2)) ;
#41502=CARTESIAN_POINT('',(-18.0758111278886,21.6113450338214,73.2)) ;
#41503=CARTESIAN_POINT('Origin',(0.,0.,73.2)) ;
#41504=CARTESIAN_POINT('',(-17.1826947828331,20.7182286887658,73.2)) ;
#41505=CARTESIAN_POINT('',(-18.9504617357995,18.9504617357995,73.2)) ;
#41506=CARTESIAN_POINT('',(-19.0211724139181,22.5567063198509,73.2)) ;
#41507=CARTESIAN_POINT('Origin',(-19.0211724139181,22.5567063198509,72.6)) ;
#41508=CARTESIAN_POINT('Ctrl Pts',(-18.0758111278886,21.6113450338214,73.2)) ;
#41509=CARTESIAN_POINT('Ctrl Pts',(-17.7794723700881,21.3150062760208,72.5910386886758)) ;
#41510=CARTESIAN_POINT('Ctrl Pts',(-17.4917855912636,21.0273194971963,72.)) ;
#41511=CARTESIAN_POINT('',(-17.1826947828331,20.7182286887658,72.6)) ;
#41512=CARTESIAN_POINT('Origin',(-18.9504617357995,18.9504617357995,72.6)) ;
#41513=CARTESIAN_POINT('Origin',(-22.6274169979695,22.6274169979695,72.6)) ;
#41514=CARTESIAN_POINT('Origin',(20.7889393668845,20.7889393668845,73.2)) ;
#41515=CARTESIAN_POINT('',(22.0372540500791,18.5017201441464,73.2)) ;
#41516=CARTESIAN_POINT('',(18.5017201441464,22.0372540500791,73.2)) ;
#41517=CARTESIAN_POINT('Origin',(0.,0.,73.2)) ;
#41518=CARTESIAN_POINT('',(24.3951839509359,20.8596500450031,73.2)) ;
#41519=CARTESIAN_POINT('',(22.5567063198509,19.0211724139181,73.2)) ;
#41520=CARTESIAN_POINT('',(20.8596500450032,24.3951839509359,73.2)) ;
#41521=CARTESIAN_POINT('',(22.6274169979695,22.6274169979695,73.2)) ;
#41522=CARTESIAN_POINT('',(19.0211724139181,22.5567063198509,73.2)) ;
#41523=CARTESIAN_POINT('Origin',(22.5567063198509,19.0211724139181,72.6)) ;
#41524=CARTESIAN_POINT('',(21.4533284625066,17.9177945565738,72.)) ;
#41525=CARTESIAN_POINT('Ctrl Pts',(21.4533284625066,17.9177945565738,72.)) ;
#41526=CARTESIAN_POINT('Ctrl Pts',(21.7410575024954,18.2055235965626,72.591231256389)) ;
#41527=CARTESIAN_POINT('Ctrl Pts',(22.0372540500791,18.5017201441464,73.2)) ;
#41528=CARTESIAN_POINT('',(24.3951839509359,20.8596500450031,72.)) ;
#41529=CARTESIAN_POINT('',(22.5567063198509,19.0211724139181,72.)) ;
#41530=CARTESIAN_POINT('',(24.3951839509359,20.8596500450031,72.6)) ;
#41531=CARTESIAN_POINT('Origin',(19.0211724139181,22.5567063198509,72.6)) ;
#41532=CARTESIAN_POINT('',(17.9177945565738,21.4533284625066,72.)) ;
#41533=CARTESIAN_POINT('Ctrl Pts',(18.5017201441464,22.0372540500791,73.2)) ;
#41534=CARTESIAN_POINT('Ctrl Pts',(18.2055235965704,21.7410575025031,72.5912312564048)) ;
#41535=CARTESIAN_POINT('Ctrl Pts',(17.9177945565738,21.4533284625066,72.)) ;
#41536=CARTESIAN_POINT('',(20.8596500450032,24.3951839509359,72.)) ;
#41537=CARTESIAN_POINT('',(20.8596500450032,24.3951839509359,72.6)) ;
#41538=CARTESIAN_POINT('',(19.0211724139181,22.5567063198509,72.)) ;
#41539=CARTESIAN_POINT('Origin',(19.0211724139181,22.5567063198509,72.6)) ;
#41540=CARTESIAN_POINT('',(17.4917855912636,21.0273194971963,72.)) ;
#41541=CARTESIAN_POINT('',(18.0758111278886,21.6113450338214,73.2)) ;
#41542=CARTESIAN_POINT('Ctrl Pts',(17.4917855912636,21.0273194971963,72.)) ;
#41543=CARTESIAN_POINT('Ctrl Pts',(17.7794723700733,21.315006276006,72.5910386886453)) ;
#41544=CARTESIAN_POINT('Ctrl Pts',(18.0758111278886,21.6113450338214,73.2)) ;
#41545=CARTESIAN_POINT('',(17.1826947828331,20.7182286887658,72.)) ;
#41546=CARTESIAN_POINT('',(19.0211724139181,22.5567063198509,72.)) ;
#41547=CARTESIAN_POINT('',(17.1826947828331,20.7182286887658,73.2)) ;
#41548=CARTESIAN_POINT('',(17.1826947828331,20.7182286887658,72.6)) ;
#41549=CARTESIAN_POINT('',(19.0211724139181,22.5567063198509,73.2)) ;
#41550=CARTESIAN_POINT('Origin',(20.7889393668845,20.7889393668845,72.)) ;
#41551=CARTESIAN_POINT('Origin',(0.,0.,72.)) ;
#41552=CARTESIAN_POINT('',(22.6274169979695,22.6274169979695,72.)) ;
#41553=CARTESIAN_POINT('Origin',(20.7889393668845,20.7889393668845,72.)) ;
#41554=CARTESIAN_POINT('',(21.0273194971963,17.4917855912636,72.)) ;
#41555=CARTESIAN_POINT('Origin',(0.,0.,72.)) ;
#41556=CARTESIAN_POINT('',(20.7182286887658,17.1826947828331,72.)) ;
#41557=CARTESIAN_POINT('',(22.5567063198509,19.0211724139181,72.)) ;
#41558=CARTESIAN_POINT('',(18.9504617357995,18.9504617357995,72.)) ;
#41559=CARTESIAN_POINT('Origin',(20.7889393668845,20.7889393668845,73.2)) ;
#41560=CARTESIAN_POINT('',(21.6113450338214,18.0758111278886,73.2)) ;
#41561=CARTESIAN_POINT('Origin',(0.,0.,73.2)) ;
#41562=CARTESIAN_POINT('',(20.7182286887658,17.1826947828331,73.2)) ;
#41563=CARTESIAN_POINT('',(18.9504617357995,18.9504617357995,73.2)) ;
#41564=CARTESIAN_POINT('',(22.5567063198509,19.0211724139181,73.2)) ;
#41565=CARTESIAN_POINT('Origin',(22.5567063198509,19.0211724139181,72.6)) ;
#41566=CARTESIAN_POINT('Ctrl Pts',(21.6113450338214,18.0758111278886,73.2)) ;
#41567=CARTESIAN_POINT('Ctrl Pts',(21.3150062760208,17.7794723700881,72.5910386886758)) ;
#41568=CARTESIAN_POINT('Ctrl Pts',(21.0273194971963,17.4917855912636,72.)) ;
#41569=CARTESIAN_POINT('',(20.7182286887658,17.1826947828331,72.6)) ;
#41570=CARTESIAN_POINT('Origin',(18.9504617357995,18.9504617357995,72.6)) ;
#41571=CARTESIAN_POINT('Origin',(22.6274169979695,22.6274169979695,72.6)) ;
#41572=CARTESIAN_POINT('Origin',(0.,0.,110.)) ;
#41573=CARTESIAN_POINT('',(-53.4,-6.53961390744687E-15,109.)) ;
#41574=CARTESIAN_POINT('Origin',(0.,0.,109.)) ;
#41575=CARTESIAN_POINT('',(-53.4,6.53961390744687E-15,109.124705882353)) ;
#41576=CARTESIAN_POINT('',(-53.4,-6.53961390744687E-15,110.)) ;
#41577=CARTESIAN_POINT('Origin',(0.,0.,109.124705882353)) ;
#41578=CARTESIAN_POINT('Origin',(0.,0.,110.)) ;
#41579=CARTESIAN_POINT('',(-53.4,6.53961390744687E-15,110.)) ;
#41580=CARTESIAN_POINT('Origin',(0.,0.,110.)) ;
#41581=CARTESIAN_POINT('',(-53.4,6.53961390744687E-15,111.)) ;
#41582=CARTESIAN_POINT('',(-53.4,-6.53961390744687E-15,110.)) ;
#41583=CARTESIAN_POINT('Origin',(0.,0.,111.)) ;
#41584=CARTESIAN_POINT('Origin',(0.,0.,109.)) ;
#41585=CARTESIAN_POINT('Origin',(0.,0.,111.)) ;
#41586=CARTESIAN_POINT('Origin',(0.,0.,79.)) ;
#41587=CARTESIAN_POINT('',(-10.9,-1.33486501107062E-15,48.)) ;
#41588=CARTESIAN_POINT('Origin',(0.,0.,48.)) ;
#41589=CARTESIAN_POINT('',(-32.15,-3.93723945925874E-15,79.)) ;
#41590=CARTESIAN_POINT('Origin',(0.,0.,79.)) ;
#41591=CARTESIAN_POINT('',(-11.5,-1.40834381901946E-15,48.)) ;
#41592=CARTESIAN_POINT('',(-32.75,-4.01071826720758E-15,79.)) ;
#41593=CARTESIAN_POINT('Origin',(0.,0.,48.)) ;
#41594=CARTESIAN_POINT('Origin',(0.,0.,48.)) ;
#50337=UNCERTAINTY_MEASURE_WITH_UNIT(LENGTH_MEASURE(0.001),#50441,
'DISTANCE_ACCURACY_VALUE',
'Maximum model space distance between geometric entities at asserted c
onnectivities') ;
#50387=UNCERTAINTY_MEASURE_WITH_UNIT(LENGTH_MEASURE(0.001),#50441,
'DISTANCE_ACCURACY_VALUE',
'Maximum model space distance between geometric entities at asserted c
onnectivities') ;
#50390=(
GEOMETRIC_REPRESENTATION_CONTEXT(3)
GLOBAL_UNCERTAINTY_ASSIGNED_CONTEXT((#50337))
GLOBAL_UNIT_ASSIGNED_CONTEXT((#50441,#50443,#50444))
REPRESENTATION_CONTEXT('','3D')
) ;
#50440=(
GEOMETRIC_REPRESENTATION_CONTEXT(3)
GLOBAL_UNCERTAINTY_ASSIGNED_CONTEXT((#50387))
GLOBAL_UNIT_ASSIGNED_CONTEXT((#50441,#50443,#50444))
REPRESENTATION_CONTEXT('','3D')
) ;
#50441=(
LENGTH_UNIT()
NAMED_UNIT(*)
SI_UNIT(.CENTI.,.METRE.)
) ;
#50443=(
NAMED_UNIT(*)
PLANE_ANGLE_UNIT()
SI_UNIT($,.RADIAN.)
) ;
#50444=(
NAMED_UNIT(*)
SI_UNIT($,.STERADIAN.)
SOLID_ANGLE_UNIT()
) ;
#50447=SHAPE_DEFINITION_REPRESENTATION(#50499,#50621) ;
#50499=PRODUCT_DEFINITION_SHAPE('',$,#50674) ;
#50621=SHAPE_REPRESENTATION('',(#29213),#50390) ;
#50671=PRODUCT_DEFINITION_CONTEXT('part definition',#50829,'design') ;
#50674=PRODUCT_DEFINITION('CONICAL_POLYETHYLENE_HOPPER',
'CONICAL_POLYETHYLENE_HOPPER',#50726,#50671) ;
#50726=PRODUCT_DEFINITION_FORMATION('',$,#50833) ;
#50829=APPLICATION_CONTEXT(
'Core Data for Automotive Mechanical Design Process') ;
#50830=PRODUCT_CONTEXT('part definition',#50829,'mechanical') ;
#50833=PRODUCT('CONICAL_POLYETHYLENE_HOPPER','CONICAL_POLYETHYLENE_HOPPER',
$,(#50830)) ;
#50884=PRESENTATION_STYLE_ASSIGNMENT((#50891)) ;
#50891=SURFACE_STYLE_USAGE(.BOTH.,#50898) ;
#50898=SURFACE_SIDE_STYLE('',(#50905)) ;
#50905=SURFACE_STYLE_FILL_AREA(#50912) ;
#50912=FILL_AREA_STYLE('Surface - Matte',(#50919)) ;
#50919=FILL_AREA_STYLE_COLOUR('Surface - Matte',#50926) ;
#50926=COLOUR_RGB('Surface - Matte', 0.72549020, 0.75294118, 0.79215686) ;
ENDSEC;
END-ISO-10303-21;
